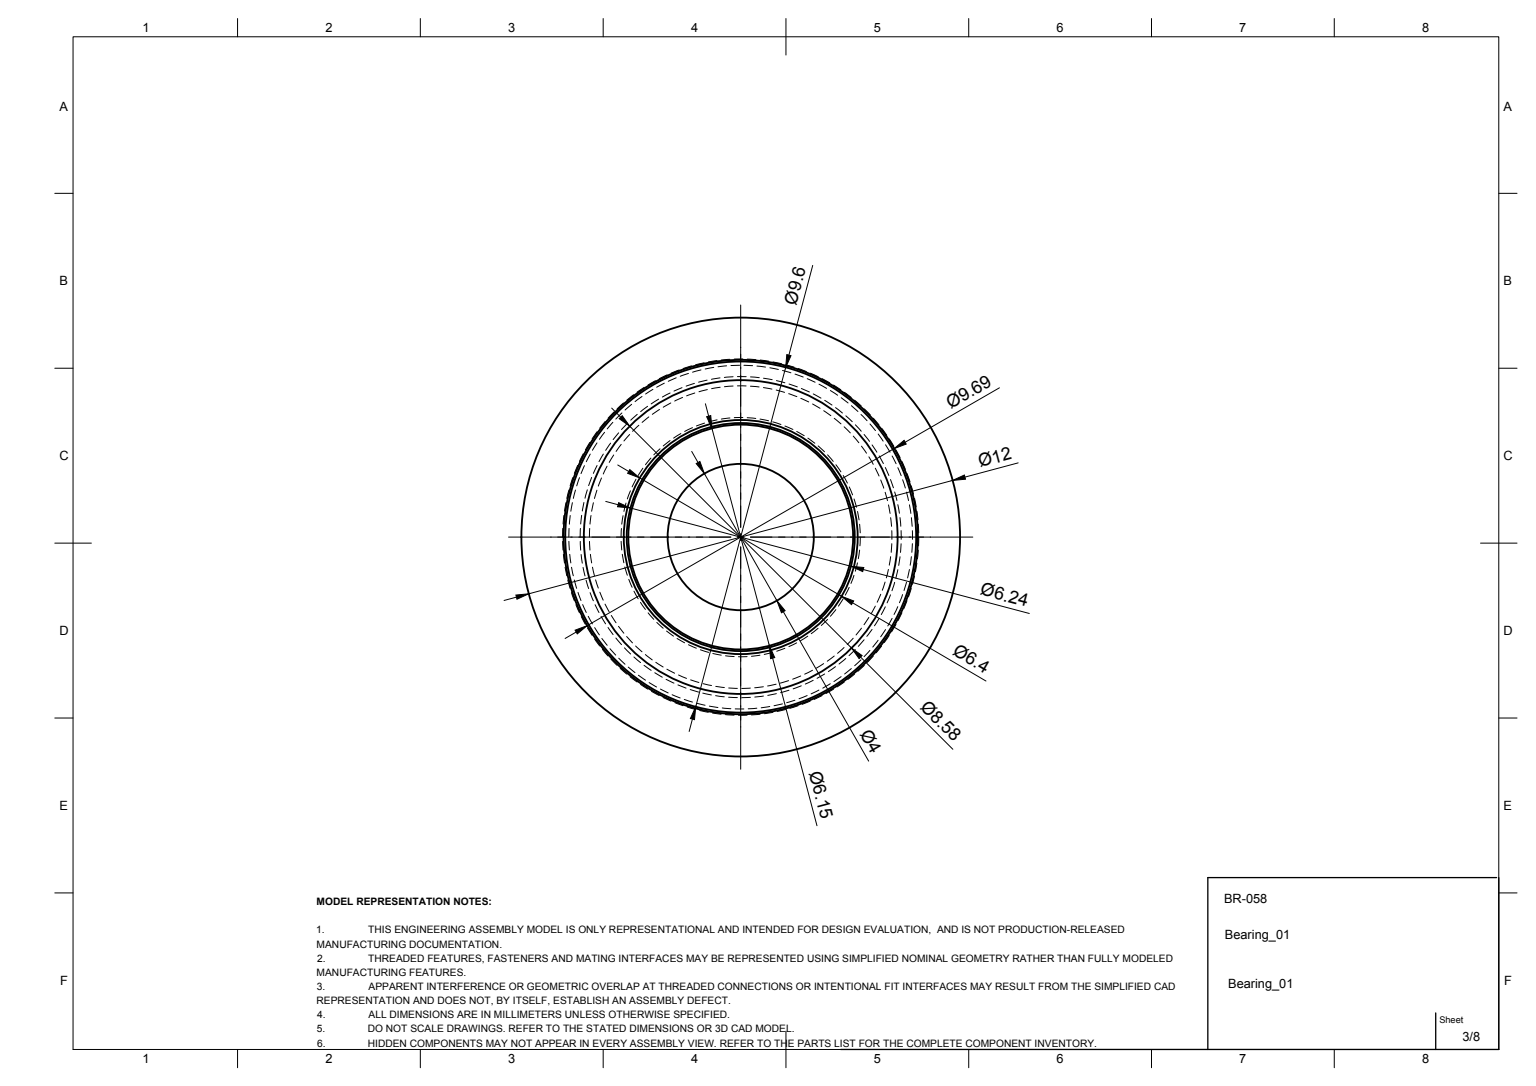
ISO-10303-21;
HEADER;
/* Generated by software containing ST-Developer
 * from STEP Tools, Inc. (www.steptools.com) 
 */

FILE_DESCRIPTION(
/* description */ (''),
/* implementation_level */ '2;1');

FILE_NAME(
/* name */ 'Bearing_01.step',
/* time_stamp */ '2026-10-12T16:07:47-07:00',
/* author */ (''),
/* organization */ (''),
/* preprocessor_version */ 'ST-DEVELOPER v20.2',
/* originating_system */ 'Autodesk Translation Framework v15.15.0.0',
/* authorisation */ '');

FILE_SCHEMA (('AUTOMOTIVE_DESIGN { 1 0 10303 214 3 1 1 }'));
ENDSEC;

DATA;
#10=MECHANICAL_DESIGN_GEOMETRIC_PRESENTATION_REPRESENTATION('',(#100,#101,#102,#103),#8779);
#43=CONICAL_SURFACE('',#5582,4.8,0.785398163397444);
#44=CONICAL_SURFACE('',#5593,4.845,0.785398163397444);
#45=CONICAL_SURFACE('',#5599,3.1184375,0.785398163397448);
#46=CONICAL_SURFACE('',#5617,3.0734375,0.785398163397448);
#47=CONICAL_SURFACE('',#5639,4.36638040039984,0.52359877559829);
#48=CONICAL_SURFACE('',#5648,4.57071796769724,1.04719755119659);
#49=CONICAL_SURFACE('',#5657,4.62071796769724,1.04719755119659);
#50=CONICAL_SURFACE('',#5666,4.27977786002139,0.52359877559829);
#51=CONICAL_SURFACE('',#5680,4.36638040039984,0.52359877559829);
#52=CONICAL_SURFACE('',#5689,4.57071796769724,1.04719755119659);
#53=CONICAL_SURFACE('',#5698,4.62071796769724,1.04719755119659);
#54=CONICAL_SURFACE('',#5707,4.27977786002139,0.52359877559829);
#56=TOROIDAL_SURFACE('',#5584,5.8,0.2);
#57=TOROIDAL_SURFACE('',#5590,5.8,0.2);
#58=TOROIDAL_SURFACE('',#5605,3.25741379310345,0.138976293103448);
#59=TOROIDAL_SURFACE('',#5611,3.25741379310345,0.138976293103448);
#60=TOROIDAL_SURFACE('',#5619,2.2,0.2);
#61=TOROIDAL_SURFACE('',#5625,2.2,0.2);
#62=TOROIDAL_SURFACE('',#5635,4.14313829631318,0.0900000000000005);
#63=TOROIDAL_SURFACE('',#5641,4.38370090847553,0.0200000000000002);
#64=TOROIDAL_SURFACE('',#5644,4.58,0.119999999999999);
#65=TOROIDAL_SURFACE('',#5650,4.51071796769724,0.12);
#66=TOROIDAL_SURFACE('',#5653,4.51071796769724,0.22);
#67=TOROIDAL_SURFACE('',#5659,4.58,0.219999999999999);
#68=TOROIDAL_SURFACE('',#5662,4.38370090847553,0.12);
#69=TOROIDAL_SURFACE('',#5676,4.14313829631318,0.0900000000000005);
#70=TOROIDAL_SURFACE('',#5682,4.38370090847553,0.0200000000000002);
#71=TOROIDAL_SURFACE('',#5685,4.58,0.119999999999999);
#72=TOROIDAL_SURFACE('',#5691,4.51071796769724,0.12);
#73=TOROIDAL_SURFACE('',#5694,4.51071796769724,0.22);
#74=TOROIDAL_SURFACE('',#5700,4.58,0.219999999999999);
#75=TOROIDAL_SURFACE('',#5703,4.38370090847553,0.12);
#86=SHAPE_REPRESENTATION_RELATIONSHIP('SRR','None',#8815,#93);
#93=ADVANCED_BREP_SHAPE_REPRESENTATION('',(#110,#111,#112,#113),#8778);
#100=STYLED_ITEM('',(#8856),#110);
#101=STYLED_ITEM('',(#8856),#111);
#102=STYLED_ITEM('',(#8856),#112);
#103=STYLED_ITEM('',(#8856),#113);
#110=MANIFOLD_SOLID_BREP('Body1',#5120);
#111=MANIFOLD_SOLID_BREP('Body2',#5121);
#112=MANIFOLD_SOLID_BREP('Body3',#5122);
#113=MANIFOLD_SOLID_BREP('Body4',#5123);
#151=FACE_BOUND('',#1015,.T.);
#152=FACE_BOUND('',#1017,.T.);
#153=FACE_BOUND('',#1019,.T.);
#154=FACE_BOUND('',#1021,.T.);
#155=FACE_BOUND('',#1033,.T.);
#156=FACE_BOUND('',#1035,.T.);
#157=FACE_BOUND('',#1037,.T.);
#158=FACE_BOUND('',#1039,.T.);
#159=FACE_BOUND('',#1053,.T.);
#160=FACE_BOUND('',#1055,.T.);
#161=FACE_BOUND('',#1057,.T.);
#162=FACE_BOUND('',#1059,.T.);
#163=FACE_BOUND('',#1061,.T.);
#164=FACE_BOUND('',#1075,.T.);
#165=FACE_BOUND('',#1077,.T.);
#166=FACE_BOUND('',#1079,.T.);
#167=FACE_BOUND('',#1081,.T.);
#168=FACE_BOUND('',#1083,.T.);
#314=CIRCLE('',#5573,4.8);
#315=CIRCLE('',#5574,4.8);
#316=CIRCLE('',#5576,4.872);
#317=CIRCLE('',#5577,4.872);
#318=CIRCLE('',#5579,4.8);
#319=CIRCLE('',#5580,4.8);
#320=CIRCLE('',#5581,4.8);
#321=CIRCLE('',#5583,4.845);
#322=CIRCLE('',#5585,6.);
#323=CIRCLE('',#5586,0.2);
#324=CIRCLE('',#5587,5.8);
#325=CIRCLE('',#5589,6.);
#326=CIRCLE('',#5591,5.8);
#327=CIRCLE('',#5592,0.2);
#328=CIRCLE('',#5594,4.845);
#329=CIRCLE('',#5600,3.1184375);
#330=CIRCLE('',#5601,3.0734375);
#331=CIRCLE('',#5602,3.1184375);
#332=CIRCLE('',#5604,3.1184375);
#333=CIRCLE('',#5606,0.138976293103448);
#334=CIRCLE('',#5607,3.2);
#335=CIRCLE('',#5609,3.272);
#336=CIRCLE('',#5610,3.272);
#337=CIRCLE('',#5612,3.2);
#338=CIRCLE('',#5613,0.138976293103448);
#339=CIRCLE('',#5614,3.1184375);
#340=CIRCLE('',#5616,3.1184375);
#341=CIRCLE('',#5618,3.0734375);
#342=CIRCLE('',#5620,2.2);
#343=CIRCLE('',#5621,0.2);
#344=CIRCLE('',#5622,2.);
#345=CIRCLE('',#5624,2.);
#346=CIRCLE('',#5626,0.2);
#347=CIRCLE('',#5627,2.2);
#348=CIRCLE('',#5633,3.2);
#349=CIRCLE('',#5634,3.2);
#350=CIRCLE('',#5636,4.22108058265378);
#351=CIRCLE('',#5637,0.0900000000000005);
#352=CIRCLE('',#5638,4.14313829631318);
#353=CIRCLE('',#5640,4.36638040039984);
#354=CIRCLE('',#5642,4.38370090847553);
#355=CIRCLE('',#5643,0.0200000000000002);
#356=CIRCLE('',#5645,4.64);
#357=CIRCLE('',#5646,0.119999999999999);
#358=CIRCLE('',#5647,4.58);
#359=CIRCLE('',#5649,4.57071796769724);
#360=CIRCLE('',#5651,4.39071796769724);
#361=CIRCLE('',#5652,0.12);
#362=CIRCLE('',#5654,4.62071796769724);
#363=CIRCLE('',#5655,0.22);
#364=CIRCLE('',#5656,4.29071796769724);
#365=CIRCLE('',#5658,4.69);
#366=CIRCLE('',#5660,4.58);
#367=CIRCLE('',#5661,0.219999999999999);
#368=CIRCLE('',#5663,4.27977786002139);
#369=CIRCLE('',#5664,0.12);
#370=CIRCLE('',#5665,4.38370090847553);
#371=CIRCLE('',#5667,4.13736479362129);
#372=CIRCLE('',#5674,3.2);
#373=CIRCLE('',#5675,3.2);
#374=CIRCLE('',#5677,4.22108058265378);
#375=CIRCLE('',#5678,0.0900000000000005);
#376=CIRCLE('',#5679,4.14313829631318);
#377=CIRCLE('',#5681,4.36638040039984);
#378=CIRCLE('',#5683,4.38370090847553);
#379=CIRCLE('',#5684,0.0200000000000002);
#380=CIRCLE('',#5686,4.64);
#381=CIRCLE('',#5687,0.119999999999999);
#382=CIRCLE('',#5688,4.58);
#383=CIRCLE('',#5690,4.57071796769724);
#384=CIRCLE('',#5692,4.39071796769724);
#385=CIRCLE('',#5693,0.12);
#386=CIRCLE('',#5695,4.62071796769724);
#387=CIRCLE('',#5696,0.22);
#388=CIRCLE('',#5697,4.29071796769724);
#389=CIRCLE('',#5699,4.69);
#390=CIRCLE('',#5701,4.58);
#391=CIRCLE('',#5702,0.219999999999999);
#392=CIRCLE('',#5704,4.27977786002139);
#393=CIRCLE('',#5705,0.12);
#394=CIRCLE('',#5706,4.38370090847553);
#395=CIRCLE('',#5708,4.13736479362129);
#465=CYLINDRICAL_SURFACE('',#5572,4.8);
#466=CYLINDRICAL_SURFACE('',#5575,4.872);
#467=CYLINDRICAL_SURFACE('',#5578,4.8);
#468=CYLINDRICAL_SURFACE('',#5588,6.);
#469=CYLINDRICAL_SURFACE('',#5603,3.1184375);
#470=CYLINDRICAL_SURFACE('',#5608,3.272);
#471=CYLINDRICAL_SURFACE('',#5615,3.1184375);
#472=CYLINDRICAL_SURFACE('',#5623,2.);
#473=CYLINDRICAL_SURFACE('',#5632,3.2);
#474=CYLINDRICAL_SURFACE('',#5673,3.2);
#692=FACE_OUTER_BOUND('',#1006,.T.);
#693=FACE_OUTER_BOUND('',#1007,.T.);
#694=FACE_OUTER_BOUND('',#1008,.T.);
#695=FACE_OUTER_BOUND('',#1009,.T.);
#696=FACE_OUTER_BOUND('',#1010,.T.);
#697=FACE_OUTER_BOUND('',#1011,.T.);
#698=FACE_OUTER_BOUND('',#1012,.T.);
#699=FACE_OUTER_BOUND('',#1013,.T.);
#700=FACE_OUTER_BOUND('',#1014,.T.);
#701=FACE_OUTER_BOUND('',#1016,.T.);
#702=FACE_OUTER_BOUND('',#1018,.T.);
#703=FACE_OUTER_BOUND('',#1020,.T.);
#704=FACE_OUTER_BOUND('',#1022,.T.);
#705=FACE_OUTER_BOUND('',#1023,.T.);
#706=FACE_OUTER_BOUND('',#1024,.T.);
#707=FACE_OUTER_BOUND('',#1025,.T.);
#708=FACE_OUTER_BOUND('',#1026,.T.);
#709=FACE_OUTER_BOUND('',#1027,.T.);
#710=FACE_OUTER_BOUND('',#1028,.T.);
#711=FACE_OUTER_BOUND('',#1029,.T.);
#712=FACE_OUTER_BOUND('',#1030,.T.);
#713=FACE_OUTER_BOUND('',#1031,.T.);
#714=FACE_OUTER_BOUND('',#1032,.T.);
#715=FACE_OUTER_BOUND('',#1034,.T.);
#716=FACE_OUTER_BOUND('',#1036,.T.);
#717=FACE_OUTER_BOUND('',#1038,.T.);
#718=FACE_OUTER_BOUND('',#1040,.T.);
#719=FACE_OUTER_BOUND('',#1041,.T.);
#720=FACE_OUTER_BOUND('',#1042,.T.);
#721=FACE_OUTER_BOUND('',#1043,.T.);
#722=FACE_OUTER_BOUND('',#1044,.T.);
#723=FACE_OUTER_BOUND('',#1045,.T.);
#724=FACE_OUTER_BOUND('',#1046,.T.);
#725=FACE_OUTER_BOUND('',#1047,.T.);
#726=FACE_OUTER_BOUND('',#1048,.T.);
#727=FACE_OUTER_BOUND('',#1049,.T.);
#728=FACE_OUTER_BOUND('',#1050,.T.);
#729=FACE_OUTER_BOUND('',#1051,.T.);
#730=FACE_OUTER_BOUND('',#1052,.T.);
#731=FACE_OUTER_BOUND('',#1054,.T.);
#732=FACE_OUTER_BOUND('',#1056,.T.);
#733=FACE_OUTER_BOUND('',#1058,.T.);
#734=FACE_OUTER_BOUND('',#1060,.T.);
#735=FACE_OUTER_BOUND('',#1062,.T.);
#736=FACE_OUTER_BOUND('',#1063,.T.);
#737=FACE_OUTER_BOUND('',#1064,.T.);
#738=FACE_OUTER_BOUND('',#1065,.T.);
#739=FACE_OUTER_BOUND('',#1066,.T.);
#740=FACE_OUTER_BOUND('',#1067,.T.);
#741=FACE_OUTER_BOUND('',#1068,.T.);
#742=FACE_OUTER_BOUND('',#1069,.T.);
#743=FACE_OUTER_BOUND('',#1070,.T.);
#744=FACE_OUTER_BOUND('',#1071,.T.);
#745=FACE_OUTER_BOUND('',#1072,.T.);
#746=FACE_OUTER_BOUND('',#1073,.T.);
#747=FACE_OUTER_BOUND('',#1074,.T.);
#748=FACE_OUTER_BOUND('',#1076,.T.);
#749=FACE_OUTER_BOUND('',#1078,.T.);
#750=FACE_OUTER_BOUND('',#1080,.T.);
#751=FACE_OUTER_BOUND('',#1082,.T.);
#1006=EDGE_LOOP('',(#4464,#4465,#4466,#4467));
#1007=EDGE_LOOP('',(#4468,#4469,#4470,#4471));
#1008=EDGE_LOOP('',(#4472,#4473,#4474,#4475,#4476));
#1009=EDGE_LOOP('',(#4477,#4478,#4479,#4480,#4481));
#1010=EDGE_LOOP('',(#4482,#4483,#4484,#4485));
#1011=EDGE_LOOP('',(#4486,#4487,#4488,#4489));
#1012=EDGE_LOOP('',(#4490,#4491,#4492,#4493));
#1013=EDGE_LOOP('',(#4494,#4495,#4496,#4497));
#1014=EDGE_LOOP('',(#4498));
#1015=EDGE_LOOP('',(#4499));
#1016=EDGE_LOOP('',(#4500));
#1017=EDGE_LOOP('',(#4501));
#1018=EDGE_LOOP('',(#4502));
#1019=EDGE_LOOP('',(#4503));
#1020=EDGE_LOOP('',(#4504));
#1021=EDGE_LOOP('',(#4505));
#1022=EDGE_LOOP('',(#4506,#4507,#4508,#4509,#4510));
#1023=EDGE_LOOP('',(#4511,#4512,#4513,#4514,#4515));
#1024=EDGE_LOOP('',(#4516,#4517,#4518,#4519));
#1025=EDGE_LOOP('',(#4520,#4521,#4522,#4523));
#1026=EDGE_LOOP('',(#4524,#4525,#4526,#4527));
#1027=EDGE_LOOP('',(#4528,#4529,#4530,#4531));
#1028=EDGE_LOOP('',(#4532,#4533,#4534,#4535));
#1029=EDGE_LOOP('',(#4536,#4537,#4538,#4539));
#1030=EDGE_LOOP('',(#4540,#4541,#4542,#4543));
#1031=EDGE_LOOP('',(#4544,#4545,#4546,#4547));
#1032=EDGE_LOOP('',(#4548));
#1033=EDGE_LOOP('',(#4549));
#1034=EDGE_LOOP('',(#4550));
#1035=EDGE_LOOP('',(#4551));
#1036=EDGE_LOOP('',(#4552));
#1037=EDGE_LOOP('',(#4553));
#1038=EDGE_LOOP('',(#4554));
#1039=EDGE_LOOP('',(#4555));
#1040=EDGE_LOOP('',(#4556,#4557,#4558,#4559));
#1041=EDGE_LOOP('',(#4560,#4561,#4562,#4563));
#1042=EDGE_LOOP('',(#4564,#4565,#4566,#4567));
#1043=EDGE_LOOP('',(#4568,#4569,#4570,#4571));
#1044=EDGE_LOOP('',(#4572,#4573,#4574,#4575));
#1045=EDGE_LOOP('',(#4576,#4577,#4578,#4579));
#1046=EDGE_LOOP('',(#4580,#4581,#4582,#4583));
#1047=EDGE_LOOP('',(#4584,#4585,#4586,#4587));
#1048=EDGE_LOOP('',(#4588,#4589,#4590,#4591));
#1049=EDGE_LOOP('',(#4592,#4593,#4594,#4595));
#1050=EDGE_LOOP('',(#4596,#4597,#4598,#4599));
#1051=EDGE_LOOP('',(#4600,#4601,#4602,#4603));
#1052=EDGE_LOOP('',(#4604));
#1053=EDGE_LOOP('',(#4605));
#1054=EDGE_LOOP('',(#4606));
#1055=EDGE_LOOP('',(#4607));
#1056=EDGE_LOOP('',(#4608));
#1057=EDGE_LOOP('',(#4609));
#1058=EDGE_LOOP('',(#4610));
#1059=EDGE_LOOP('',(#4611));
#1060=EDGE_LOOP('',(#4612));
#1061=EDGE_LOOP('',(#4613));
#1062=EDGE_LOOP('',(#4614,#4615,#4616,#4617));
#1063=EDGE_LOOP('',(#4618,#4619,#4620,#4621));
#1064=EDGE_LOOP('',(#4622,#4623,#4624,#4625));
#1065=EDGE_LOOP('',(#4626,#4627,#4628,#4629));
#1066=EDGE_LOOP('',(#4630,#4631,#4632,#4633));
#1067=EDGE_LOOP('',(#4634,#4635,#4636,#4637));
#1068=EDGE_LOOP('',(#4638,#4639,#4640,#4641));
#1069=EDGE_LOOP('',(#4642,#4643,#4644,#4645));
#1070=EDGE_LOOP('',(#4646,#4647,#4648,#4649));
#1071=EDGE_LOOP('',(#4650,#4651,#4652,#4653));
#1072=EDGE_LOOP('',(#4654,#4655,#4656,#4657));
#1073=EDGE_LOOP('',(#4658,#4659,#4660,#4661));
#1074=EDGE_LOOP('',(#4662));
#1075=EDGE_LOOP('',(#4663));
#1076=EDGE_LOOP('',(#4664));
#1077=EDGE_LOOP('',(#4665));
#1078=EDGE_LOOP('',(#4666));
#1079=EDGE_LOOP('',(#4667));
#1080=EDGE_LOOP('',(#4668));
#1081=EDGE_LOOP('',(#4669));
#1082=EDGE_LOOP('',(#4670));
#1083=EDGE_LOOP('',(#4671));
#1547=LINE('',#8532,#2032);
#1548=LINE('',#8538,#2033);
#1549=LINE('',#8546,#2034);
#1550=LINE('',#8550,#2035);
#1551=LINE('',#8561,#2036);
#1552=LINE('',#8568,#2037);
#1553=LINE('',#8579,#2038);
#1554=LINE('',#8584,#2039);
#1555=LINE('',#8594,#2040);
#1556=LINE('',#8604,#2041);
#1557=LINE('',#8608,#2042);
#1558=LINE('',#8618,#2043);
#1559=LINE('',#8632,#2044);
#1560=LINE('',#8643,#2045);
#1561=LINE('',#8657,#2046);
#1562=LINE('',#8671,#2047);
#1563=LINE('',#8685,#2048);
#1564=LINE('',#8695,#2049);
#1565=LINE('',#8706,#2050);
#1566=LINE('',#8720,#2051);
#1567=LINE('',#8734,#2052);
#1568=LINE('',#8748,#2053);
#2032=VECTOR('',#6929,4.8);
#2033=VECTOR('',#6936,4.872);
#2034=VECTOR('',#6945,4.8);
#2035=VECTOR('',#6950,4.8);
#2036=VECTOR('',#6965,6.);
#2037=VECTOR('',#6974,4.845);
#2038=VECTOR('',#6989,3.1184375);
#2039=VECTOR('',#6996,3.1184375);
#2040=VECTOR('',#7009,3.272);
#2041=VECTOR('',#7022,3.1184375);
#2042=VECTOR('',#7027,3.0734375);
#2043=VECTOR('',#7040,2.);
#2044=VECTOR('',#7061,3.2);
#2045=VECTOR('',#7076,4.36638040039984);
#2046=VECTOR('',#7095,4.57071796769724);
#2047=VECTOR('',#7114,4.62071796769724);
#2048=VECTOR('',#7133,4.27977786002139);
#2049=VECTOR('',#7148,3.2);
#2050=VECTOR('',#7163,4.36638040039984);
#2051=VECTOR('',#7182,4.57071796769724);
#2052=VECTOR('',#7201,4.62071796769724);
#2053=VECTOR('',#7220,4.27977786002139);
#2462=VERTEX_POINT('',#8529);
#2463=VERTEX_POINT('',#8531);
#2464=VERTEX_POINT('',#8535);
#2465=VERTEX_POINT('',#8537);
#2466=VERTEX_POINT('',#8541);
#2467=VERTEX_POINT('',#8542);
#2468=VERTEX_POINT('',#8545);
#2469=VERTEX_POINT('',#8549);
#2470=VERTEX_POINT('',#8553);
#2471=VERTEX_POINT('',#8555);
#2472=VERTEX_POINT('',#8559);
#2473=VERTEX_POINT('',#8563);
#2474=VERTEX_POINT('',#8567);
#2475=VERTEX_POINT('',#8575);
#2476=VERTEX_POINT('',#8576);
#2477=VERTEX_POINT('',#8578);
#2478=VERTEX_POINT('',#8583);
#2479=VERTEX_POINT('',#8587);
#2480=VERTEX_POINT('',#8591);
#2481=VERTEX_POINT('',#8593);
#2482=VERTEX_POINT('',#8597);
#2483=VERTEX_POINT('',#8599);
#2484=VERTEX_POINT('',#8603);
#2485=VERTEX_POINT('',#8607);
#2486=VERTEX_POINT('',#8611);
#2487=VERTEX_POINT('',#8613);
#2488=VERTEX_POINT('',#8617);
#2489=VERTEX_POINT('',#8621);
#2490=VERTEX_POINT('',#8629);
#2491=VERTEX_POINT('',#8631);
#2492=VERTEX_POINT('',#8635);
#2493=VERTEX_POINT('',#8637);
#2494=VERTEX_POINT('',#8641);
#2495=VERTEX_POINT('',#8645);
#2496=VERTEX_POINT('',#8649);
#2497=VERTEX_POINT('',#8651);
#2498=VERTEX_POINT('',#8655);
#2499=VERTEX_POINT('',#8659);
#2500=VERTEX_POINT('',#8663);
#2501=VERTEX_POINT('',#8665);
#2502=VERTEX_POINT('',#8669);
#2503=VERTEX_POINT('',#8673);
#2504=VERTEX_POINT('',#8677);
#2505=VERTEX_POINT('',#8679);
#2506=VERTEX_POINT('',#8683);
#2507=VERTEX_POINT('',#8692);
#2508=VERTEX_POINT('',#8694);
#2509=VERTEX_POINT('',#8698);
#2510=VERTEX_POINT('',#8700);
#2511=VERTEX_POINT('',#8704);
#2512=VERTEX_POINT('',#8708);
#2513=VERTEX_POINT('',#8712);
#2514=VERTEX_POINT('',#8714);
#2515=VERTEX_POINT('',#8718);
#2516=VERTEX_POINT('',#8722);
#2517=VERTEX_POINT('',#8726);
#2518=VERTEX_POINT('',#8728);
#2519=VERTEX_POINT('',#8732);
#2520=VERTEX_POINT('',#8736);
#2521=VERTEX_POINT('',#8740);
#2522=VERTEX_POINT('',#8742);
#2523=VERTEX_POINT('',#8746);
#3136=EDGE_CURVE('',#2462,#2462,#314,.T.);
#3137=EDGE_CURVE('',#2462,#2463,#1547,.T.);
#3138=EDGE_CURVE('',#2463,#2463,#315,.T.);
#3139=EDGE_CURVE('',#2464,#2464,#316,.T.);
#3140=EDGE_CURVE('',#2464,#2465,#1548,.T.);
#3141=EDGE_CURVE('',#2465,#2465,#317,.T.);
#3142=EDGE_CURVE('',#2466,#2467,#318,.T.);
#3143=EDGE_CURVE('',#2467,#2466,#319,.T.);
#3144=EDGE_CURVE('',#2467,#2468,#1549,.T.);
#3145=EDGE_CURVE('',#2468,#2468,#320,.T.);
#3146=EDGE_CURVE('',#2466,#2469,#1550,.T.);
#3147=EDGE_CURVE('',#2469,#2469,#321,.T.);
#3148=EDGE_CURVE('',#2470,#2470,#322,.T.);
#3149=EDGE_CURVE('',#2470,#2471,#323,.T.);
#3150=EDGE_CURVE('',#2471,#2471,#324,.T.);
#3151=EDGE_CURVE('',#2472,#2472,#325,.T.);
#3152=EDGE_CURVE('',#2472,#2470,#1551,.T.);
#3153=EDGE_CURVE('',#2473,#2473,#326,.T.);
#3154=EDGE_CURVE('',#2473,#2472,#327,.T.);
#3155=EDGE_CURVE('',#2463,#2474,#1552,.T.);
#3156=EDGE_CURVE('',#2474,#2474,#328,.T.);
#3157=EDGE_CURVE('',#2475,#2476,#329,.T.);
#3158=EDGE_CURVE('',#2476,#2477,#1553,.T.);
#3159=EDGE_CURVE('',#2477,#2477,#330,.T.);
#3160=EDGE_CURVE('',#2476,#2475,#331,.T.);
#3161=EDGE_CURVE('',#2475,#2478,#1554,.T.);
#3162=EDGE_CURVE('',#2478,#2478,#332,.T.);
#3163=EDGE_CURVE('',#2478,#2479,#333,.T.);
#3164=EDGE_CURVE('',#2479,#2479,#334,.T.);
#3165=EDGE_CURVE('',#2480,#2480,#335,.T.);
#3166=EDGE_CURVE('',#2480,#2481,#1555,.T.);
#3167=EDGE_CURVE('',#2481,#2481,#336,.T.);
#3168=EDGE_CURVE('',#2482,#2482,#337,.T.);
#3169=EDGE_CURVE('',#2482,#2483,#338,.T.);
#3170=EDGE_CURVE('',#2483,#2483,#339,.T.);
#3171=EDGE_CURVE('',#2483,#2484,#1556,.T.);
#3172=EDGE_CURVE('',#2484,#2484,#340,.T.);
#3173=EDGE_CURVE('',#2484,#2485,#1557,.T.);
#3174=EDGE_CURVE('',#2485,#2485,#341,.T.);
#3175=EDGE_CURVE('',#2486,#2486,#342,.T.);
#3176=EDGE_CURVE('',#2486,#2487,#343,.T.);
#3177=EDGE_CURVE('',#2487,#2487,#344,.T.);
#3178=EDGE_CURVE('',#2487,#2488,#1558,.T.);
#3179=EDGE_CURVE('',#2488,#2488,#345,.T.);
#3180=EDGE_CURVE('',#2488,#2489,#346,.T.);
#3181=EDGE_CURVE('',#2489,#2489,#347,.T.);
#3182=EDGE_CURVE('',#2490,#2490,#348,.T.);
#3183=EDGE_CURVE('',#2490,#2491,#1559,.T.);
#3184=EDGE_CURVE('',#2491,#2491,#349,.T.);
#3185=EDGE_CURVE('',#2492,#2492,#350,.T.);
#3186=EDGE_CURVE('',#2492,#2493,#351,.T.);
#3187=EDGE_CURVE('',#2493,#2493,#352,.T.);
#3188=EDGE_CURVE('',#2494,#2494,#353,.T.);
#3189=EDGE_CURVE('',#2494,#2492,#1560,.T.);
#3190=EDGE_CURVE('',#2495,#2495,#354,.T.);
#3191=EDGE_CURVE('',#2495,#2494,#355,.T.);
#3192=EDGE_CURVE('',#2496,#2496,#356,.T.);
#3193=EDGE_CURVE('',#2496,#2497,#357,.T.);
#3194=EDGE_CURVE('',#2497,#2497,#358,.T.);
#3195=EDGE_CURVE('',#2498,#2498,#359,.T.);
#3196=EDGE_CURVE('',#2498,#2496,#1561,.T.);
#3197=EDGE_CURVE('',#2499,#2499,#360,.T.);
#3198=EDGE_CURVE('',#2499,#2498,#361,.T.);
#3199=EDGE_CURVE('',#2500,#2500,#362,.T.);
#3200=EDGE_CURVE('',#2500,#2501,#363,.T.);
#3201=EDGE_CURVE('',#2501,#2501,#364,.T.);
#3202=EDGE_CURVE('',#2502,#2502,#365,.T.);
#3203=EDGE_CURVE('',#2502,#2500,#1562,.T.);
#3204=EDGE_CURVE('',#2503,#2503,#366,.T.);
#3205=EDGE_CURVE('',#2503,#2502,#367,.T.);
#3206=EDGE_CURVE('',#2504,#2504,#368,.T.);
#3207=EDGE_CURVE('',#2504,#2505,#369,.T.);
#3208=EDGE_CURVE('',#2505,#2505,#370,.T.);
#3209=EDGE_CURVE('',#2506,#2506,#371,.T.);
#3210=EDGE_CURVE('',#2506,#2504,#1563,.T.);
#3211=EDGE_CURVE('',#2507,#2507,#372,.T.);
#3212=EDGE_CURVE('',#2507,#2508,#1564,.T.);
#3213=EDGE_CURVE('',#2508,#2508,#373,.T.);
#3214=EDGE_CURVE('',#2509,#2509,#374,.T.);
#3215=EDGE_CURVE('',#2509,#2510,#375,.T.);
#3216=EDGE_CURVE('',#2510,#2510,#376,.T.);
#3217=EDGE_CURVE('',#2511,#2511,#377,.T.);
#3218=EDGE_CURVE('',#2511,#2509,#1565,.T.);
#3219=EDGE_CURVE('',#2512,#2512,#378,.T.);
#3220=EDGE_CURVE('',#2512,#2511,#379,.T.);
#3221=EDGE_CURVE('',#2513,#2513,#380,.T.);
#3222=EDGE_CURVE('',#2513,#2514,#381,.T.);
#3223=EDGE_CURVE('',#2514,#2514,#382,.T.);
#3224=EDGE_CURVE('',#2515,#2515,#383,.T.);
#3225=EDGE_CURVE('',#2515,#2513,#1566,.T.);
#3226=EDGE_CURVE('',#2516,#2516,#384,.T.);
#3227=EDGE_CURVE('',#2516,#2515,#385,.T.);
#3228=EDGE_CURVE('',#2517,#2517,#386,.T.);
#3229=EDGE_CURVE('',#2517,#2518,#387,.T.);
#3230=EDGE_CURVE('',#2518,#2518,#388,.T.);
#3231=EDGE_CURVE('',#2519,#2519,#389,.T.);
#3232=EDGE_CURVE('',#2519,#2517,#1567,.T.);
#3233=EDGE_CURVE('',#2520,#2520,#390,.T.);
#3234=EDGE_CURVE('',#2520,#2519,#391,.T.);
#3235=EDGE_CURVE('',#2521,#2521,#392,.T.);
#3236=EDGE_CURVE('',#2521,#2522,#393,.T.);
#3237=EDGE_CURVE('',#2522,#2522,#394,.T.);
#3238=EDGE_CURVE('',#2523,#2523,#395,.T.);
#3239=EDGE_CURVE('',#2523,#2521,#1568,.T.);
#4464=ORIENTED_EDGE('',*,*,#3136,.F.);
#4465=ORIENTED_EDGE('',*,*,#3137,.T.);
#4466=ORIENTED_EDGE('',*,*,#3138,.T.);
#4467=ORIENTED_EDGE('',*,*,#3137,.F.);
#4468=ORIENTED_EDGE('',*,*,#3139,.F.);
#4469=ORIENTED_EDGE('',*,*,#3140,.T.);
#4470=ORIENTED_EDGE('',*,*,#3141,.T.);
#4471=ORIENTED_EDGE('',*,*,#3140,.F.);
#4472=ORIENTED_EDGE('',*,*,#3142,.F.);
#4473=ORIENTED_EDGE('',*,*,#3143,.F.);
#4474=ORIENTED_EDGE('',*,*,#3144,.T.);
#4475=ORIENTED_EDGE('',*,*,#3145,.T.);
#4476=ORIENTED_EDGE('',*,*,#3144,.F.);
#4477=ORIENTED_EDGE('',*,*,#3142,.T.);
#4478=ORIENTED_EDGE('',*,*,#3143,.T.);
#4479=ORIENTED_EDGE('',*,*,#3146,.T.);
#4480=ORIENTED_EDGE('',*,*,#3147,.F.);
#4481=ORIENTED_EDGE('',*,*,#3146,.F.);
#4482=ORIENTED_EDGE('',*,*,#3148,.F.);
#4483=ORIENTED_EDGE('',*,*,#3149,.T.);
#4484=ORIENTED_EDGE('',*,*,#3150,.T.);
#4485=ORIENTED_EDGE('',*,*,#3149,.F.);
#4486=ORIENTED_EDGE('',*,*,#3151,.F.);
#4487=ORIENTED_EDGE('',*,*,#3152,.T.);
#4488=ORIENTED_EDGE('',*,*,#3148,.T.);
#4489=ORIENTED_EDGE('',*,*,#3152,.F.);
#4490=ORIENTED_EDGE('',*,*,#3153,.F.);
#4491=ORIENTED_EDGE('',*,*,#3154,.T.);
#4492=ORIENTED_EDGE('',*,*,#3151,.T.);
#4493=ORIENTED_EDGE('',*,*,#3154,.F.);
#4494=ORIENTED_EDGE('',*,*,#3138,.F.);
#4495=ORIENTED_EDGE('',*,*,#3155,.T.);
#4496=ORIENTED_EDGE('',*,*,#3156,.T.);
#4497=ORIENTED_EDGE('',*,*,#3155,.F.);
#4498=ORIENTED_EDGE('',*,*,#3153,.T.);
#4499=ORIENTED_EDGE('',*,*,#3156,.F.);
#4500=ORIENTED_EDGE('',*,*,#3150,.F.);
#4501=ORIENTED_EDGE('',*,*,#3147,.T.);
#4502=ORIENTED_EDGE('',*,*,#3139,.T.);
#4503=ORIENTED_EDGE('',*,*,#3145,.F.);
#4504=ORIENTED_EDGE('',*,*,#3141,.F.);
#4505=ORIENTED_EDGE('',*,*,#3136,.T.);
#4506=ORIENTED_EDGE('',*,*,#3157,.T.);
#4507=ORIENTED_EDGE('',*,*,#3158,.T.);
#4508=ORIENTED_EDGE('',*,*,#3159,.F.);
#4509=ORIENTED_EDGE('',*,*,#3158,.F.);
#4510=ORIENTED_EDGE('',*,*,#3160,.T.);
#4511=ORIENTED_EDGE('',*,*,#3157,.F.);
#4512=ORIENTED_EDGE('',*,*,#3161,.T.);
#4513=ORIENTED_EDGE('',*,*,#3162,.T.);
#4514=ORIENTED_EDGE('',*,*,#3161,.F.);
#4515=ORIENTED_EDGE('',*,*,#3160,.F.);
#4516=ORIENTED_EDGE('',*,*,#3162,.F.);
#4517=ORIENTED_EDGE('',*,*,#3163,.T.);
#4518=ORIENTED_EDGE('',*,*,#3164,.T.);
#4519=ORIENTED_EDGE('',*,*,#3163,.F.);
#4520=ORIENTED_EDGE('',*,*,#3165,.F.);
#4521=ORIENTED_EDGE('',*,*,#3166,.T.);
#4522=ORIENTED_EDGE('',*,*,#3167,.T.);
#4523=ORIENTED_EDGE('',*,*,#3166,.F.);
#4524=ORIENTED_EDGE('',*,*,#3168,.F.);
#4525=ORIENTED_EDGE('',*,*,#3169,.T.);
#4526=ORIENTED_EDGE('',*,*,#3170,.T.);
#4527=ORIENTED_EDGE('',*,*,#3169,.F.);
#4528=ORIENTED_EDGE('',*,*,#3170,.F.);
#4529=ORIENTED_EDGE('',*,*,#3171,.T.);
#4530=ORIENTED_EDGE('',*,*,#3172,.T.);
#4531=ORIENTED_EDGE('',*,*,#3171,.F.);
#4532=ORIENTED_EDGE('',*,*,#3172,.F.);
#4533=ORIENTED_EDGE('',*,*,#3173,.T.);
#4534=ORIENTED_EDGE('',*,*,#3174,.T.);
#4535=ORIENTED_EDGE('',*,*,#3173,.F.);
#4536=ORIENTED_EDGE('',*,*,#3175,.F.);
#4537=ORIENTED_EDGE('',*,*,#3176,.T.);
#4538=ORIENTED_EDGE('',*,*,#3177,.T.);
#4539=ORIENTED_EDGE('',*,*,#3176,.F.);
#4540=ORIENTED_EDGE('',*,*,#3177,.F.);
#4541=ORIENTED_EDGE('',*,*,#3178,.T.);
#4542=ORIENTED_EDGE('',*,*,#3179,.T.);
#4543=ORIENTED_EDGE('',*,*,#3178,.F.);
#4544=ORIENTED_EDGE('',*,*,#3179,.F.);
#4545=ORIENTED_EDGE('',*,*,#3180,.T.);
#4546=ORIENTED_EDGE('',*,*,#3181,.T.);
#4547=ORIENTED_EDGE('',*,*,#3180,.F.);
#4548=ORIENTED_EDGE('',*,*,#3174,.F.);
#4549=ORIENTED_EDGE('',*,*,#3175,.T.);
#4550=ORIENTED_EDGE('',*,*,#3167,.F.);
#4551=ORIENTED_EDGE('',*,*,#3168,.T.);
#4552=ORIENTED_EDGE('',*,*,#3165,.T.);
#4553=ORIENTED_EDGE('',*,*,#3164,.F.);
#4554=ORIENTED_EDGE('',*,*,#3159,.T.);
#4555=ORIENTED_EDGE('',*,*,#3181,.F.);
#4556=ORIENTED_EDGE('',*,*,#3182,.F.);
#4557=ORIENTED_EDGE('',*,*,#3183,.T.);
#4558=ORIENTED_EDGE('',*,*,#3184,.T.);
#4559=ORIENTED_EDGE('',*,*,#3183,.F.);
#4560=ORIENTED_EDGE('',*,*,#3185,.F.);
#4561=ORIENTED_EDGE('',*,*,#3186,.T.);
#4562=ORIENTED_EDGE('',*,*,#3187,.T.);
#4563=ORIENTED_EDGE('',*,*,#3186,.F.);
#4564=ORIENTED_EDGE('',*,*,#3188,.F.);
#4565=ORIENTED_EDGE('',*,*,#3189,.T.);
#4566=ORIENTED_EDGE('',*,*,#3185,.T.);
#4567=ORIENTED_EDGE('',*,*,#3189,.F.);
#4568=ORIENTED_EDGE('',*,*,#3190,.F.);
#4569=ORIENTED_EDGE('',*,*,#3191,.T.);
#4570=ORIENTED_EDGE('',*,*,#3188,.T.);
#4571=ORIENTED_EDGE('',*,*,#3191,.F.);
#4572=ORIENTED_EDGE('',*,*,#3192,.F.);
#4573=ORIENTED_EDGE('',*,*,#3193,.T.);
#4574=ORIENTED_EDGE('',*,*,#3194,.T.);
#4575=ORIENTED_EDGE('',*,*,#3193,.F.);
#4576=ORIENTED_EDGE('',*,*,#3195,.F.);
#4577=ORIENTED_EDGE('',*,*,#3196,.T.);
#4578=ORIENTED_EDGE('',*,*,#3192,.T.);
#4579=ORIENTED_EDGE('',*,*,#3196,.F.);
#4580=ORIENTED_EDGE('',*,*,#3197,.F.);
#4581=ORIENTED_EDGE('',*,*,#3198,.T.);
#4582=ORIENTED_EDGE('',*,*,#3195,.T.);
#4583=ORIENTED_EDGE('',*,*,#3198,.F.);
#4584=ORIENTED_EDGE('',*,*,#3199,.F.);
#4585=ORIENTED_EDGE('',*,*,#3200,.T.);
#4586=ORIENTED_EDGE('',*,*,#3201,.T.);
#4587=ORIENTED_EDGE('',*,*,#3200,.F.);
#4588=ORIENTED_EDGE('',*,*,#3202,.F.);
#4589=ORIENTED_EDGE('',*,*,#3203,.T.);
#4590=ORIENTED_EDGE('',*,*,#3199,.T.);
#4591=ORIENTED_EDGE('',*,*,#3203,.F.);
#4592=ORIENTED_EDGE('',*,*,#3204,.F.);
#4593=ORIENTED_EDGE('',*,*,#3205,.T.);
#4594=ORIENTED_EDGE('',*,*,#3202,.T.);
#4595=ORIENTED_EDGE('',*,*,#3205,.F.);
#4596=ORIENTED_EDGE('',*,*,#3206,.F.);
#4597=ORIENTED_EDGE('',*,*,#3207,.T.);
#4598=ORIENTED_EDGE('',*,*,#3208,.T.);
#4599=ORIENTED_EDGE('',*,*,#3207,.F.);
#4600=ORIENTED_EDGE('',*,*,#3209,.F.);
#4601=ORIENTED_EDGE('',*,*,#3210,.T.);
#4602=ORIENTED_EDGE('',*,*,#3206,.T.);
#4603=ORIENTED_EDGE('',*,*,#3210,.F.);
#4604=ORIENTED_EDGE('',*,*,#3209,.T.);
#4605=ORIENTED_EDGE('',*,*,#3184,.F.);
#4606=ORIENTED_EDGE('',*,*,#3204,.T.);
#4607=ORIENTED_EDGE('',*,*,#3208,.F.);
#4608=ORIENTED_EDGE('',*,*,#3197,.T.);
#4609=ORIENTED_EDGE('',*,*,#3201,.F.);
#4610=ORIENTED_EDGE('',*,*,#3194,.F.);
#4611=ORIENTED_EDGE('',*,*,#3190,.T.);
#4612=ORIENTED_EDGE('',*,*,#3187,.F.);
#4613=ORIENTED_EDGE('',*,*,#3182,.T.);
#4614=ORIENTED_EDGE('',*,*,#3211,.T.);
#4615=ORIENTED_EDGE('',*,*,#3212,.T.);
#4616=ORIENTED_EDGE('',*,*,#3213,.F.);
#4617=ORIENTED_EDGE('',*,*,#3212,.F.);
#4618=ORIENTED_EDGE('',*,*,#3214,.T.);
#4619=ORIENTED_EDGE('',*,*,#3215,.T.);
#4620=ORIENTED_EDGE('',*,*,#3216,.F.);
#4621=ORIENTED_EDGE('',*,*,#3215,.F.);
#4622=ORIENTED_EDGE('',*,*,#3217,.T.);
#4623=ORIENTED_EDGE('',*,*,#3218,.T.);
#4624=ORIENTED_EDGE('',*,*,#3214,.F.);
#4625=ORIENTED_EDGE('',*,*,#3218,.F.);
#4626=ORIENTED_EDGE('',*,*,#3219,.T.);
#4627=ORIENTED_EDGE('',*,*,#3220,.T.);
#4628=ORIENTED_EDGE('',*,*,#3217,.F.);
#4629=ORIENTED_EDGE('',*,*,#3220,.F.);
#4630=ORIENTED_EDGE('',*,*,#3221,.T.);
#4631=ORIENTED_EDGE('',*,*,#3222,.T.);
#4632=ORIENTED_EDGE('',*,*,#3223,.F.);
#4633=ORIENTED_EDGE('',*,*,#3222,.F.);
#4634=ORIENTED_EDGE('',*,*,#3224,.T.);
#4635=ORIENTED_EDGE('',*,*,#3225,.T.);
#4636=ORIENTED_EDGE('',*,*,#3221,.F.);
#4637=ORIENTED_EDGE('',*,*,#3225,.F.);
#4638=ORIENTED_EDGE('',*,*,#3226,.T.);
#4639=ORIENTED_EDGE('',*,*,#3227,.T.);
#4640=ORIENTED_EDGE('',*,*,#3224,.F.);
#4641=ORIENTED_EDGE('',*,*,#3227,.F.);
#4642=ORIENTED_EDGE('',*,*,#3228,.T.);
#4643=ORIENTED_EDGE('',*,*,#3229,.T.);
#4644=ORIENTED_EDGE('',*,*,#3230,.F.);
#4645=ORIENTED_EDGE('',*,*,#3229,.F.);
#4646=ORIENTED_EDGE('',*,*,#3231,.T.);
#4647=ORIENTED_EDGE('',*,*,#3232,.T.);
#4648=ORIENTED_EDGE('',*,*,#3228,.F.);
#4649=ORIENTED_EDGE('',*,*,#3232,.F.);
#4650=ORIENTED_EDGE('',*,*,#3233,.T.);
#4651=ORIENTED_EDGE('',*,*,#3234,.T.);
#4652=ORIENTED_EDGE('',*,*,#3231,.F.);
#4653=ORIENTED_EDGE('',*,*,#3234,.F.);
#4654=ORIENTED_EDGE('',*,*,#3235,.T.);
#4655=ORIENTED_EDGE('',*,*,#3236,.T.);
#4656=ORIENTED_EDGE('',*,*,#3237,.F.);
#4657=ORIENTED_EDGE('',*,*,#3236,.F.);
#4658=ORIENTED_EDGE('',*,*,#3238,.T.);
#4659=ORIENTED_EDGE('',*,*,#3239,.T.);
#4660=ORIENTED_EDGE('',*,*,#3235,.F.);
#4661=ORIENTED_EDGE('',*,*,#3239,.F.);
#4662=ORIENTED_EDGE('',*,*,#3238,.F.);
#4663=ORIENTED_EDGE('',*,*,#3213,.T.);
#4664=ORIENTED_EDGE('',*,*,#3233,.F.);
#4665=ORIENTED_EDGE('',*,*,#3237,.T.);
#4666=ORIENTED_EDGE('',*,*,#3226,.F.);
#4667=ORIENTED_EDGE('',*,*,#3230,.T.);
#4668=ORIENTED_EDGE('',*,*,#3223,.T.);
#4669=ORIENTED_EDGE('',*,*,#3219,.F.);
#4670=ORIENTED_EDGE('',*,*,#3216,.T.);
#4671=ORIENTED_EDGE('',*,*,#3211,.F.);
#4819=PLANE('',#5595);
#4820=PLANE('',#5596);
#4821=PLANE('',#5597);
#4822=PLANE('',#5598);
#4823=PLANE('',#5628);
#4824=PLANE('',#5629);
#4825=PLANE('',#5630);
#4826=PLANE('',#5631);
#4827=PLANE('',#5668);
#4828=PLANE('',#5669);
#4829=PLANE('',#5670);
#4830=PLANE('',#5671);
#4831=PLANE('',#5672);
#4832=PLANE('',#5709);
#4833=PLANE('',#5710);
#4834=PLANE('',#5711);
#4835=PLANE('',#5712);
#4836=PLANE('',#5713);
#5054=ADVANCED_FACE('',(#692),#465,.F.);
#5055=ADVANCED_FACE('',(#693),#466,.F.);
#5056=ADVANCED_FACE('',(#694),#467,.F.);
#5057=ADVANCED_FACE('',(#695),#43,.F.);
#5058=ADVANCED_FACE('',(#696),#56,.T.);
#5059=ADVANCED_FACE('',(#697),#468,.T.);
#5060=ADVANCED_FACE('',(#698),#57,.T.);
#5061=ADVANCED_FACE('',(#699),#44,.F.);
#5062=ADVANCED_FACE('',(#700,#151),#4819,.F.);
#5063=ADVANCED_FACE('',(#701,#152),#4820,.F.);
#5064=ADVANCED_FACE('',(#702,#153),#4821,.F.);
#5065=ADVANCED_FACE('',(#703,#154),#4822,.F.);
#5066=ADVANCED_FACE('',(#704),#45,.T.);
#5067=ADVANCED_FACE('',(#705),#469,.T.);
#5068=ADVANCED_FACE('',(#706),#58,.F.);
#5069=ADVANCED_FACE('',(#707),#470,.T.);
#5070=ADVANCED_FACE('',(#708),#59,.F.);
#5071=ADVANCED_FACE('',(#709),#471,.T.);
#5072=ADVANCED_FACE('',(#710),#46,.T.);
#5073=ADVANCED_FACE('',(#711),#60,.T.);
#5074=ADVANCED_FACE('',(#712),#472,.F.);
#5075=ADVANCED_FACE('',(#713),#61,.T.);
#5076=ADVANCED_FACE('',(#714,#155),#4823,.F.);
#5077=ADVANCED_FACE('',(#715,#156),#4824,.F.);
#5078=ADVANCED_FACE('',(#716,#157),#4825,.F.);
#5079=ADVANCED_FACE('',(#717,#158),#4826,.F.);
#5080=ADVANCED_FACE('',(#718),#473,.F.);
#5081=ADVANCED_FACE('',(#719),#62,.T.);
#5082=ADVANCED_FACE('',(#720),#47,.T.);
#5083=ADVANCED_FACE('',(#721),#63,.F.);
#5084=ADVANCED_FACE('',(#722),#64,.F.);
#5085=ADVANCED_FACE('',(#723),#48,.F.);
#5086=ADVANCED_FACE('',(#724),#65,.F.);
#5087=ADVANCED_FACE('',(#725),#66,.T.);
#5088=ADVANCED_FACE('',(#726),#49,.T.);
#5089=ADVANCED_FACE('',(#727),#67,.T.);
#5090=ADVANCED_FACE('',(#728),#68,.T.);
#5091=ADVANCED_FACE('',(#729),#50,.F.);
#5092=ADVANCED_FACE('',(#730,#159),#4827,.F.);
#5093=ADVANCED_FACE('',(#731,#160),#4828,.F.);
#5094=ADVANCED_FACE('',(#732,#161),#4829,.T.);
#5095=ADVANCED_FACE('',(#733,#162),#4830,.T.);
#5096=ADVANCED_FACE('',(#734,#163),#4831,.T.);
#5097=ADVANCED_FACE('',(#735),#474,.F.);
#5098=ADVANCED_FACE('',(#736),#69,.T.);
#5099=ADVANCED_FACE('',(#737),#51,.T.);
#5100=ADVANCED_FACE('',(#738),#70,.F.);
#5101=ADVANCED_FACE('',(#739),#71,.F.);
#5102=ADVANCED_FACE('',(#740),#52,.F.);
#5103=ADVANCED_FACE('',(#741),#72,.F.);
#5104=ADVANCED_FACE('',(#742),#73,.T.);
#5105=ADVANCED_FACE('',(#743),#53,.T.);
#5106=ADVANCED_FACE('',(#744),#74,.T.);
#5107=ADVANCED_FACE('',(#745),#75,.T.);
#5108=ADVANCED_FACE('',(#746),#54,.F.);
#5109=ADVANCED_FACE('',(#747,#164),#4832,.F.);
#5110=ADVANCED_FACE('',(#748,#165),#4833,.F.);
#5111=ADVANCED_FACE('',(#749,#166),#4834,.T.);
#5112=ADVANCED_FACE('',(#750,#167),#4835,.T.);
#5113=ADVANCED_FACE('',(#751,#168),#4836,.T.);
#5120=CLOSED_SHELL('',(#5054,#5055,#5056,#5057,#5058,#5059,#5060,#5061,
#5062,#5063,#5064,#5065));
#5121=CLOSED_SHELL('',(#5066,#5067,#5068,#5069,#5070,#5071,#5072,#5073,
#5074,#5075,#5076,#5077,#5078,#5079));
#5122=CLOSED_SHELL('',(#5080,#5081,#5082,#5083,#5084,#5085,#5086,#5087,
#5088,#5089,#5090,#5091,#5092,#5093,#5094,#5095,#5096));
#5123=CLOSED_SHELL('',(#5097,#5098,#5099,#5100,#5101,#5102,#5103,#5104,
#5105,#5106,#5107,#5108,#5109,#5110,#5111,#5112,#5113));
#5571=AXIS2_PLACEMENT_3D('',#8527,#6923,#6924);
#5572=AXIS2_PLACEMENT_3D('',#8528,#6925,#6926);
#5573=AXIS2_PLACEMENT_3D('',#8530,#6927,#6928);
#5574=AXIS2_PLACEMENT_3D('',#8533,#6930,#6931);
#5575=AXIS2_PLACEMENT_3D('',#8534,#6932,#6933);
#5576=AXIS2_PLACEMENT_3D('',#8536,#6934,#6935);
#5577=AXIS2_PLACEMENT_3D('',#8539,#6937,#6938);
#5578=AXIS2_PLACEMENT_3D('',#8540,#6939,#6940);
#5579=AXIS2_PLACEMENT_3D('',#8543,#6941,#6942);
#5580=AXIS2_PLACEMENT_3D('',#8544,#6943,#6944);
#5581=AXIS2_PLACEMENT_3D('',#8547,#6946,#6947);
#5582=AXIS2_PLACEMENT_3D('',#8548,#6948,#6949);
#5583=AXIS2_PLACEMENT_3D('',#8551,#6951,#6952);
#5584=AXIS2_PLACEMENT_3D('',#8552,#6953,#6954);
#5585=AXIS2_PLACEMENT_3D('',#8554,#6955,#6956);
#5586=AXIS2_PLACEMENT_3D('',#8556,#6957,#6958);
#5587=AXIS2_PLACEMENT_3D('',#8557,#6959,#6960);
#5588=AXIS2_PLACEMENT_3D('',#8558,#6961,#6962);
#5589=AXIS2_PLACEMENT_3D('',#8560,#6963,#6964);
#5590=AXIS2_PLACEMENT_3D('',#8562,#6966,#6967);
#5591=AXIS2_PLACEMENT_3D('',#8564,#6968,#6969);
#5592=AXIS2_PLACEMENT_3D('',#8565,#6970,#6971);
#5593=AXIS2_PLACEMENT_3D('',#8566,#6972,#6973);
#5594=AXIS2_PLACEMENT_3D('',#8569,#6975,#6976);
#5595=AXIS2_PLACEMENT_3D('',#8570,#6977,#6978);
#5596=AXIS2_PLACEMENT_3D('',#8571,#6979,#6980);
#5597=AXIS2_PLACEMENT_3D('',#8572,#6981,#6982);
#5598=AXIS2_PLACEMENT_3D('',#8573,#6983,#6984);
#5599=AXIS2_PLACEMENT_3D('',#8574,#6985,#6986);
#5600=AXIS2_PLACEMENT_3D('',#8577,#6987,#6988);
#5601=AXIS2_PLACEMENT_3D('',#8580,#6990,#6991);
#5602=AXIS2_PLACEMENT_3D('',#8581,#6992,#6993);
#5603=AXIS2_PLACEMENT_3D('',#8582,#6994,#6995);
#5604=AXIS2_PLACEMENT_3D('',#8585,#6997,#6998);
#5605=AXIS2_PLACEMENT_3D('',#8586,#6999,#7000);
#5606=AXIS2_PLACEMENT_3D('',#8588,#7001,#7002);
#5607=AXIS2_PLACEMENT_3D('',#8589,#7003,#7004);
#5608=AXIS2_PLACEMENT_3D('',#8590,#7005,#7006);
#5609=AXIS2_PLACEMENT_3D('',#8592,#7007,#7008);
#5610=AXIS2_PLACEMENT_3D('',#8595,#7010,#7011);
#5611=AXIS2_PLACEMENT_3D('',#8596,#7012,#7013);
#5612=AXIS2_PLACEMENT_3D('',#8598,#7014,#7015);
#5613=AXIS2_PLACEMENT_3D('',#8600,#7016,#7017);
#5614=AXIS2_PLACEMENT_3D('',#8601,#7018,#7019);
#5615=AXIS2_PLACEMENT_3D('',#8602,#7020,#7021);
#5616=AXIS2_PLACEMENT_3D('',#8605,#7023,#7024);
#5617=AXIS2_PLACEMENT_3D('',#8606,#7025,#7026);
#5618=AXIS2_PLACEMENT_3D('',#8609,#7028,#7029);
#5619=AXIS2_PLACEMENT_3D('',#8610,#7030,#7031);
#5620=AXIS2_PLACEMENT_3D('',#8612,#7032,#7033);
#5621=AXIS2_PLACEMENT_3D('',#8614,#7034,#7035);
#5622=AXIS2_PLACEMENT_3D('',#8615,#7036,#7037);
#5623=AXIS2_PLACEMENT_3D('',#8616,#7038,#7039);
#5624=AXIS2_PLACEMENT_3D('',#8619,#7041,#7042);
#5625=AXIS2_PLACEMENT_3D('',#8620,#7043,#7044);
#5626=AXIS2_PLACEMENT_3D('',#8622,#7045,#7046);
#5627=AXIS2_PLACEMENT_3D('',#8623,#7047,#7048);
#5628=AXIS2_PLACEMENT_3D('',#8624,#7049,#7050);
#5629=AXIS2_PLACEMENT_3D('',#8625,#7051,#7052);
#5630=AXIS2_PLACEMENT_3D('',#8626,#7053,#7054);
#5631=AXIS2_PLACEMENT_3D('',#8627,#7055,#7056);
#5632=AXIS2_PLACEMENT_3D('',#8628,#7057,#7058);
#5633=AXIS2_PLACEMENT_3D('',#8630,#7059,#7060);
#5634=AXIS2_PLACEMENT_3D('',#8633,#7062,#7063);
#5635=AXIS2_PLACEMENT_3D('',#8634,#7064,#7065);
#5636=AXIS2_PLACEMENT_3D('',#8636,#7066,#7067);
#5637=AXIS2_PLACEMENT_3D('',#8638,#7068,#7069);
#5638=AXIS2_PLACEMENT_3D('',#8639,#7070,#7071);
#5639=AXIS2_PLACEMENT_3D('',#8640,#7072,#7073);
#5640=AXIS2_PLACEMENT_3D('',#8642,#7074,#7075);
#5641=AXIS2_PLACEMENT_3D('',#8644,#7077,#7078);
#5642=AXIS2_PLACEMENT_3D('',#8646,#7079,#7080);
#5643=AXIS2_PLACEMENT_3D('',#8647,#7081,#7082);
#5644=AXIS2_PLACEMENT_3D('',#8648,#7083,#7084);
#5645=AXIS2_PLACEMENT_3D('',#8650,#7085,#7086);
#5646=AXIS2_PLACEMENT_3D('',#8652,#7087,#7088);
#5647=AXIS2_PLACEMENT_3D('',#8653,#7089,#7090);
#5648=AXIS2_PLACEMENT_3D('',#8654,#7091,#7092);
#5649=AXIS2_PLACEMENT_3D('',#8656,#7093,#7094);
#5650=AXIS2_PLACEMENT_3D('',#8658,#7096,#7097);
#5651=AXIS2_PLACEMENT_3D('',#8660,#7098,#7099);
#5652=AXIS2_PLACEMENT_3D('',#8661,#7100,#7101);
#5653=AXIS2_PLACEMENT_3D('',#8662,#7102,#7103);
#5654=AXIS2_PLACEMENT_3D('',#8664,#7104,#7105);
#5655=AXIS2_PLACEMENT_3D('',#8666,#7106,#7107);
#5656=AXIS2_PLACEMENT_3D('',#8667,#7108,#7109);
#5657=AXIS2_PLACEMENT_3D('',#8668,#7110,#7111);
#5658=AXIS2_PLACEMENT_3D('',#8670,#7112,#7113);
#5659=AXIS2_PLACEMENT_3D('',#8672,#7115,#7116);
#5660=AXIS2_PLACEMENT_3D('',#8674,#7117,#7118);
#5661=AXIS2_PLACEMENT_3D('',#8675,#7119,#7120);
#5662=AXIS2_PLACEMENT_3D('',#8676,#7121,#7122);
#5663=AXIS2_PLACEMENT_3D('',#8678,#7123,#7124);
#5664=AXIS2_PLACEMENT_3D('',#8680,#7125,#7126);
#5665=AXIS2_PLACEMENT_3D('',#8681,#7127,#7128);
#5666=AXIS2_PLACEMENT_3D('',#8682,#7129,#7130);
#5667=AXIS2_PLACEMENT_3D('',#8684,#7131,#7132);
#5668=AXIS2_PLACEMENT_3D('',#8686,#7134,#7135);
#5669=AXIS2_PLACEMENT_3D('',#8687,#7136,#7137);
#5670=AXIS2_PLACEMENT_3D('',#8688,#7138,#7139);
#5671=AXIS2_PLACEMENT_3D('',#8689,#7140,#7141);
#5672=AXIS2_PLACEMENT_3D('',#8690,#7142,#7143);
#5673=AXIS2_PLACEMENT_3D('',#8691,#7144,#7145);
#5674=AXIS2_PLACEMENT_3D('',#8693,#7146,#7147);
#5675=AXIS2_PLACEMENT_3D('',#8696,#7149,#7150);
#5676=AXIS2_PLACEMENT_3D('',#8697,#7151,#7152);
#5677=AXIS2_PLACEMENT_3D('',#8699,#7153,#7154);
#5678=AXIS2_PLACEMENT_3D('',#8701,#7155,#7156);
#5679=AXIS2_PLACEMENT_3D('',#8702,#7157,#7158);
#5680=AXIS2_PLACEMENT_3D('',#8703,#7159,#7160);
#5681=AXIS2_PLACEMENT_3D('',#8705,#7161,#7162);
#5682=AXIS2_PLACEMENT_3D('',#8707,#7164,#7165);
#5683=AXIS2_PLACEMENT_3D('',#8709,#7166,#7167);
#5684=AXIS2_PLACEMENT_3D('',#8710,#7168,#7169);
#5685=AXIS2_PLACEMENT_3D('',#8711,#7170,#7171);
#5686=AXIS2_PLACEMENT_3D('',#8713,#7172,#7173);
#5687=AXIS2_PLACEMENT_3D('',#8715,#7174,#7175);
#5688=AXIS2_PLACEMENT_3D('',#8716,#7176,#7177);
#5689=AXIS2_PLACEMENT_3D('',#8717,#7178,#7179);
#5690=AXIS2_PLACEMENT_3D('',#8719,#7180,#7181);
#5691=AXIS2_PLACEMENT_3D('',#8721,#7183,#7184);
#5692=AXIS2_PLACEMENT_3D('',#8723,#7185,#7186);
#5693=AXIS2_PLACEMENT_3D('',#8724,#7187,#7188);
#5694=AXIS2_PLACEMENT_3D('',#8725,#7189,#7190);
#5695=AXIS2_PLACEMENT_3D('',#8727,#7191,#7192);
#5696=AXIS2_PLACEMENT_3D('',#8729,#7193,#7194);
#5697=AXIS2_PLACEMENT_3D('',#8730,#7195,#7196);
#5698=AXIS2_PLACEMENT_3D('',#8731,#7197,#7198);
#5699=AXIS2_PLACEMENT_3D('',#8733,#7199,#7200);
#5700=AXIS2_PLACEMENT_3D('',#8735,#7202,#7203);
#5701=AXIS2_PLACEMENT_3D('',#8737,#7204,#7205);
#5702=AXIS2_PLACEMENT_3D('',#8738,#7206,#7207);
#5703=AXIS2_PLACEMENT_3D('',#8739,#7208,#7209);
#5704=AXIS2_PLACEMENT_3D('',#8741,#7210,#7211);
#5705=AXIS2_PLACEMENT_3D('',#8743,#7212,#7213);
#5706=AXIS2_PLACEMENT_3D('',#8744,#7214,#7215);
#5707=AXIS2_PLACEMENT_3D('',#8745,#7216,#7217);
#5708=AXIS2_PLACEMENT_3D('',#8747,#7218,#7219);
#5709=AXIS2_PLACEMENT_3D('',#8749,#7221,#7222);
#5710=AXIS2_PLACEMENT_3D('',#8750,#7223,#7224);
#5711=AXIS2_PLACEMENT_3D('',#8751,#7225,#7226);
#5712=AXIS2_PLACEMENT_3D('',#8752,#7227,#7228);
#5713=AXIS2_PLACEMENT_3D('',#8753,#7229,#7230);
#6923=DIRECTION('axis',(0.,0.,1.));
#6924=DIRECTION('refdir',(1.,0.,0.));
#6925=DIRECTION('center_axis',(-1.,-1.83697019872103E-16,0.));
#6926=DIRECTION('ref_axis',(1.83697019872103E-16,-1.,0.));
#6927=DIRECTION('center_axis',(-1.,-1.83697019872103E-16,0.));
#6928=DIRECTION('ref_axis',(1.83697019872103E-16,-1.,0.));
#6929=DIRECTION('',(-1.,-1.83697019872103E-16,0.));
#6930=DIRECTION('center_axis',(-1.,-1.83697019872103E-16,0.));
#6931=DIRECTION('ref_axis',(1.83697019872103E-16,-1.,0.));
#6932=DIRECTION('center_axis',(-1.,-1.83697019872103E-16,0.));
#6933=DIRECTION('ref_axis',(1.83697019872103E-16,-1.,0.));
#6934=DIRECTION('center_axis',(-1.,-1.83697019872103E-16,0.));
#6935=DIRECTION('ref_axis',(1.83697019872103E-16,-1.,0.));
#6936=DIRECTION('',(-1.,-1.83697019872103E-16,0.));
#6937=DIRECTION('center_axis',(-1.,-1.83697019872103E-16,0.));
#6938=DIRECTION('ref_axis',(1.83697019872103E-16,-1.,0.));
#6939=DIRECTION('center_axis',(-1.,-1.83697019872103E-16,0.));
#6940=DIRECTION('ref_axis',(1.83697019872103E-16,-1.,0.));
#6941=DIRECTION('center_axis',(-1.,-1.83697019872103E-16,0.));
#6942=DIRECTION('ref_axis',(1.83697019872103E-16,-1.,0.));
#6943=DIRECTION('center_axis',(-1.,-1.83697019872103E-16,0.));
#6944=DIRECTION('ref_axis',(1.83697019872103E-16,-1.,0.));
#6945=DIRECTION('',(-1.,-1.83697019872103E-16,0.));
#6946=DIRECTION('center_axis',(-1.,-1.83697019872103E-16,0.));
#6947=DIRECTION('ref_axis',(1.83697019872103E-16,-1.,0.));
#6948=DIRECTION('center_axis',(1.,1.83697019872103E-16,0.));
#6949=DIRECTION('ref_axis',(-1.83697019872103E-16,1.,0.));
#6950=DIRECTION('',(0.707106781186551,-0.707106781186544,-8.6595605623549E-17));
#6951=DIRECTION('center_axis',(-1.,-1.83697019872103E-16,0.));
#6952=DIRECTION('ref_axis',(1.83697019872103E-16,-1.,0.));
#6953=DIRECTION('center_axis',(-1.,-1.83697019872103E-16,0.));
#6954=DIRECTION('ref_axis',(1.85037170770859E-16,-1.,0.));
#6955=DIRECTION('center_axis',(-1.,-1.83697019872103E-16,0.));
#6956=DIRECTION('ref_axis',(1.83697019872103E-16,-1.,0.));
#6957=DIRECTION('center_axis',(2.24963967399279E-32,-1.22464679914735E-16,
-1.));
#6958=DIRECTION('ref_axis',(-1.85037170770859E-16,1.,-1.22464679914735E-16));
#6959=DIRECTION('center_axis',(-1.,-1.83697019872103E-16,0.));
#6960=DIRECTION('ref_axis',(1.83697019872103E-16,-1.,0.));
#6961=DIRECTION('center_axis',(-1.,-1.83697019872103E-16,0.));
#6962=DIRECTION('ref_axis',(1.83697019872103E-16,-1.,0.));
#6963=DIRECTION('center_axis',(-1.,-1.83697019872103E-16,0.));
#6964=DIRECTION('ref_axis',(1.83697019872103E-16,-1.,0.));
#6965=DIRECTION('',(1.,1.83697019872103E-16,0.));
#6966=DIRECTION('center_axis',(-1.,-1.83697019872103E-16,0.));
#6967=DIRECTION('ref_axis',(1.85037170770859E-16,-1.,0.));
#6968=DIRECTION('center_axis',(-1.,-1.83697019872103E-16,0.));
#6969=DIRECTION('ref_axis',(1.83697019872103E-16,-1.,0.));
#6970=DIRECTION('center_axis',(2.24963967399279E-32,-1.22464679914735E-16,
-1.));
#6971=DIRECTION('ref_axis',(-1.85037170770859E-16,1.,-1.22464679914735E-16));
#6972=DIRECTION('center_axis',(-1.,-1.83697019872103E-16,0.));
#6973=DIRECTION('ref_axis',(1.83697019872103E-16,-1.,0.));
#6974=DIRECTION('',(-0.707106781186551,0.707106781186544,-8.6595605623549E-17));
#6975=DIRECTION('center_axis',(-1.,-1.83697019872103E-16,0.));
#6976=DIRECTION('ref_axis',(1.83697019872103E-16,-1.,0.));
#6977=DIRECTION('center_axis',(1.,1.83697019872103E-16,0.));
#6978=DIRECTION('ref_axis',(-1.83697019872103E-16,1.,0.));
#6979=DIRECTION('center_axis',(-1.,-1.83697019872103E-16,0.));
#6980=DIRECTION('ref_axis',(1.83697019872103E-16,-1.,0.));
#6981=DIRECTION('center_axis',(1.,1.83697019872103E-16,0.));
#6982=DIRECTION('ref_axis',(-1.83697019872103E-16,1.,0.));
#6983=DIRECTION('center_axis',(-1.,-1.83697019872103E-16,0.));
#6984=DIRECTION('ref_axis',(1.83697019872103E-16,-1.,0.));
#6985=DIRECTION('center_axis',(1.,1.83697019872103E-16,0.));
#6986=DIRECTION('ref_axis',(-1.83697019872103E-16,1.,0.));
#6987=DIRECTION('center_axis',(-1.,-1.83697019872103E-16,0.));
#6988=DIRECTION('ref_axis',(1.83697019872103E-16,-1.,0.));
#6989=DIRECTION('',(-0.707106781186548,0.707106781186547,8.65956056235493E-17));
#6990=DIRECTION('center_axis',(-1.,-1.83697019872103E-16,0.));
#6991=DIRECTION('ref_axis',(1.83697019872103E-16,-1.,0.));
#6992=DIRECTION('center_axis',(-1.,-1.83697019872103E-16,0.));
#6993=DIRECTION('ref_axis',(1.83697019872103E-16,-1.,0.));
#6994=DIRECTION('center_axis',(-1.,-1.83697019872103E-16,0.));
#6995=DIRECTION('ref_axis',(1.83697019872103E-16,-1.,0.));
#6996=DIRECTION('',(1.,1.83697019872103E-16,0.));
#6997=DIRECTION('center_axis',(-1.,-1.83697019872103E-16,0.));
#6998=DIRECTION('ref_axis',(1.83697019872103E-16,-1.,0.));
#6999=DIRECTION('center_axis',(-1.,-1.83697019872103E-16,0.));
#7000=DIRECTION('ref_axis',(1.96129949112834E-16,-1.,0.));
#7001=DIRECTION('center_axis',(-2.24963967399279E-32,1.22464679914735E-16,
1.));
#7002=DIRECTION('ref_axis',(-1.63441624260695E-16,1.,-1.22464679914735E-16));
#7003=DIRECTION('center_axis',(-1.,-1.83697019872103E-16,0.));
#7004=DIRECTION('ref_axis',(1.83697019872103E-16,-1.,0.));
#7005=DIRECTION('center_axis',(-1.,-1.83697019872103E-16,0.));
#7006=DIRECTION('ref_axis',(1.83697019872103E-16,-1.,0.));
#7007=DIRECTION('center_axis',(-1.,-1.83697019872103E-16,0.));
#7008=DIRECTION('ref_axis',(1.83697019872103E-16,-1.,0.));
#7009=DIRECTION('',(1.,1.83697019872103E-16,0.));
#7010=DIRECTION('center_axis',(-1.,-1.83697019872103E-16,0.));
#7011=DIRECTION('ref_axis',(1.83697019872103E-16,-1.,0.));
#7012=DIRECTION('center_axis',(-1.,-1.83697019872103E-16,0.));
#7013=DIRECTION('ref_axis',(1.96129949112834E-16,-1.,0.));
#7014=DIRECTION('center_axis',(-1.,-1.83697019872103E-16,0.));
#7015=DIRECTION('ref_axis',(1.83697019872103E-16,-1.,0.));
#7016=DIRECTION('center_axis',(-2.24963967399279E-32,1.22464679914735E-16,
1.));
#7017=DIRECTION('ref_axis',(-1.63441624260695E-16,1.,-1.22464679914735E-16));
#7018=DIRECTION('center_axis',(-1.,-1.83697019872103E-16,0.));
#7019=DIRECTION('ref_axis',(1.83697019872103E-16,-1.,0.));
#7020=DIRECTION('center_axis',(-1.,-1.83697019872103E-16,0.));
#7021=DIRECTION('ref_axis',(1.83697019872103E-16,-1.,0.));
#7022=DIRECTION('',(1.,1.83697019872103E-16,0.));
#7023=DIRECTION('center_axis',(-1.,-1.83697019872103E-16,0.));
#7024=DIRECTION('ref_axis',(1.83697019872103E-16,-1.,0.));
#7025=DIRECTION('center_axis',(-1.,-1.83697019872103E-16,0.));
#7026=DIRECTION('ref_axis',(1.83697019872103E-16,-1.,0.));
#7027=DIRECTION('',(0.707106781186548,-0.707106781186547,8.65956056235493E-17));
#7028=DIRECTION('center_axis',(-1.,-1.83697019872103E-16,0.));
#7029=DIRECTION('ref_axis',(1.83697019872103E-16,-1.,0.));
#7030=DIRECTION('center_axis',(-1.,-1.83697019872103E-16,0.));
#7031=DIRECTION('ref_axis',(1.85037170770859E-16,-1.,0.));
#7032=DIRECTION('center_axis',(-1.,-1.83697019872103E-16,0.));
#7033=DIRECTION('ref_axis',(1.83697019872103E-16,-1.,0.));
#7034=DIRECTION('center_axis',(2.24963967399279E-32,-1.22464679914735E-16,
-1.));
#7035=DIRECTION('ref_axis',(-2.31296463463574E-16,1.,-1.22464679914735E-16));
#7036=DIRECTION('center_axis',(-1.,-1.83697019872103E-16,0.));
#7037=DIRECTION('ref_axis',(1.83697019872103E-16,-1.,0.));
#7038=DIRECTION('center_axis',(-1.,-1.83697019872103E-16,0.));
#7039=DIRECTION('ref_axis',(1.83697019872103E-16,-1.,0.));
#7040=DIRECTION('',(-1.,-1.83697019872103E-16,0.));
#7041=DIRECTION('center_axis',(-1.,-1.83697019872103E-16,0.));
#7042=DIRECTION('ref_axis',(1.83697019872103E-16,-1.,0.));
#7043=DIRECTION('center_axis',(-1.,-1.83697019872103E-16,0.));
#7044=DIRECTION('ref_axis',(1.85037170770859E-16,-1.,0.));
#7045=DIRECTION('center_axis',(2.24963967399279E-32,-1.22464679914735E-16,
-1.));
#7046=DIRECTION('ref_axis',(-2.31296463463574E-16,1.,-1.22464679914735E-16));
#7047=DIRECTION('center_axis',(-1.,-1.83697019872103E-16,0.));
#7048=DIRECTION('ref_axis',(1.83697019872103E-16,-1.,0.));
#7049=DIRECTION('center_axis',(-1.,-1.83697019872103E-16,0.));
#7050=DIRECTION('ref_axis',(1.83697019872103E-16,-1.,0.));
#7051=DIRECTION('center_axis',(-1.,-1.83697019872103E-16,0.));
#7052=DIRECTION('ref_axis',(1.83697019872103E-16,-1.,0.));
#7053=DIRECTION('center_axis',(1.,1.83697019872103E-16,0.));
#7054=DIRECTION('ref_axis',(-1.83697019872103E-16,1.,0.));
#7055=DIRECTION('center_axis',(1.,1.83697019872103E-16,0.));
#7056=DIRECTION('ref_axis',(-1.83697019872103E-16,1.,0.));
#7057=DIRECTION('center_axis',(-1.,-1.83697019872103E-16,0.));
#7058=DIRECTION('ref_axis',(1.83697019872103E-16,-1.,0.));
#7059=DIRECTION('center_axis',(-1.,-1.83697019872103E-16,0.));
#7060=DIRECTION('ref_axis',(1.83697019872103E-16,-1.,0.));
#7061=DIRECTION('',(-1.,-1.83697019872103E-16,0.));
#7062=DIRECTION('center_axis',(-1.,-1.83697019872103E-16,0.));
#7063=DIRECTION('ref_axis',(1.83697019872103E-16,-1.,0.));
#7064=DIRECTION('center_axis',(-1.,-1.83697019872103E-16,0.));
#7065=DIRECTION('ref_axis',(1.57361694361665E-16,-1.,0.));
#7066=DIRECTION('center_axis',(-1.,-1.83697019872103E-16,0.));
#7067=DIRECTION('ref_axis',(1.83697019872103E-16,-1.,0.));
#7068=DIRECTION('center_axis',(2.24963967399279E-32,-1.22464679914735E-16,
-1.));
#7069=DIRECTION('ref_axis',(-1.96702117952081E-16,1.,-1.22464679914735E-16));
#7070=DIRECTION('center_axis',(-1.,-1.83697019872103E-16,0.));
#7071=DIRECTION('ref_axis',(1.83697019872103E-16,-1.,0.));
#7072=DIRECTION('center_axis',(-1.,-1.83697019872103E-16,0.));
#7073=DIRECTION('ref_axis',(1.83697019872103E-16,-1.,0.));
#7074=DIRECTION('center_axis',(-1.,-1.83697019872103E-16,0.));
#7075=DIRECTION('ref_axis',(1.83697019872103E-16,-1.,0.));
#7076=DIRECTION('',(0.866025403784443,-0.499999999999992,6.12323399573667E-17));
#7077=DIRECTION('center_axis',(-1.,-1.83697019872103E-16,0.));
#7078=DIRECTION('ref_axis',(2.01689087919369E-16,-1.,0.));
#7079=DIRECTION('center_axis',(-1.,-1.83697019872103E-16,0.));
#7080=DIRECTION('ref_axis',(1.83697019872103E-16,-1.,0.));
#7081=DIRECTION('center_axis',(-2.24963967399279E-32,1.22464679914735E-16,
1.));
#7082=DIRECTION('ref_axis',(-1.89083519924408E-16,1.,-1.22464679914735E-16));
#7083=DIRECTION('center_axis',(-1.,-1.83697019872103E-16,0.));
#7084=DIRECTION('ref_axis',(1.88974131851091E-16,-1.,0.));
#7085=DIRECTION('center_axis',(-1.,-1.83697019872103E-16,0.));
#7086=DIRECTION('ref_axis',(1.83697019872103E-16,-1.,0.));
#7087=DIRECTION('center_axis',(-2.24963967399279E-32,1.22464679914735E-16,
1.));
#7088=DIRECTION('ref_axis',(-1.77163248610397E-16,1.,-1.22464679914735E-16));
#7089=DIRECTION('center_axis',(-1.,-1.83697019872103E-16,0.));
#7090=DIRECTION('ref_axis',(1.83697019872103E-16,-1.,0.));
#7091=DIRECTION('center_axis',(-1.,-1.83697019872103E-16,0.));
#7092=DIRECTION('ref_axis',(1.83697019872103E-16,-1.,0.));
#7093=DIRECTION('center_axis',(-1.,-1.83697019872103E-16,0.));
#7094=DIRECTION('ref_axis',(1.83697019872103E-16,-1.,0.));
#7095=DIRECTION('',(-0.500000000000007,0.866025403784435,-1.0605752387249E-16));
#7096=DIRECTION('center_axis',(-1.,-1.83697019872103E-16,0.));
#7097=DIRECTION('ref_axis',(1.91801449774277E-16,-1.,0.));
#7098=DIRECTION('center_axis',(-1.,-1.83697019872103E-16,0.));
#7099=DIRECTION('ref_axis',(1.83697019872103E-16,-1.,0.));
#7100=DIRECTION('center_axis',(-2.24963967399279E-32,1.22464679914735E-16,
1.));
#7101=DIRECTION('ref_axis',(-1.79813859163385E-16,1.,-1.22464679914735E-16));
#7102=DIRECTION('center_axis',(-1.,-1.83697019872103E-16,0.));
#7103=DIRECTION('ref_axis',(1.87747066251861E-16,-1.,0.));
#7104=DIRECTION('center_axis',(-1.,-1.83697019872103E-16,0.));
#7105=DIRECTION('ref_axis',(1.83697019872103E-16,-1.,0.));
#7106=DIRECTION('center_axis',(2.24963967399279E-32,-1.22464679914735E-16,
-1.));
#7107=DIRECTION('ref_axis',(-1.7601287461112E-16,1.,-1.22464679914735E-16));
#7108=DIRECTION('center_axis',(-1.,-1.83697019872103E-16,0.));
#7109=DIRECTION('ref_axis',(1.83697019872103E-16,-1.,0.));
#7110=DIRECTION('center_axis',(-1.,-1.83697019872103E-16,0.));
#7111=DIRECTION('ref_axis',(1.83697019872103E-16,-1.,0.));
#7112=DIRECTION('center_axis',(-1.,-1.83697019872103E-16,0.));
#7113=DIRECTION('ref_axis',(1.83697019872103E-16,-1.,0.));
#7114=DIRECTION('',(0.500000000000007,-0.866025403784435,1.0605752387249E-16));
#7115=DIRECTION('center_axis',(-1.,-1.83697019872103E-16,0.));
#7116=DIRECTION('ref_axis',(1.85037170770859E-16,-1.,0.));
#7117=DIRECTION('center_axis',(-1.,-1.83697019872103E-16,0.));
#7118=DIRECTION('ref_axis',(1.83697019872103E-16,-1.,0.));
#7119=DIRECTION('center_axis',(2.24963967399279E-32,-1.22464679914735E-16,
-1.));
#7120=DIRECTION('ref_axis',(-1.73472347597681E-16,1.,-1.22464679914735E-16));
#7121=DIRECTION('center_axis',(-1.,-1.83697019872103E-16,0.));
#7122=DIRECTION('ref_axis',(1.97210791246963E-16,-1.,0.));
#7123=DIRECTION('center_axis',(-1.,-1.83697019872103E-16,0.));
#7124=DIRECTION('ref_axis',(1.83697019872103E-16,-1.,0.));
#7125=DIRECTION('center_axis',(2.24963967399279E-32,-1.22464679914735E-16,
-1.));
#7126=DIRECTION('ref_axis',(-1.84885116794028E-16,1.,-1.22464679914735E-16));
#7127=DIRECTION('center_axis',(-1.,-1.83697019872103E-16,0.));
#7128=DIRECTION('ref_axis',(1.83697019872103E-16,-1.,0.));
#7129=DIRECTION('center_axis',(-1.,-1.83697019872103E-16,0.));
#7130=DIRECTION('ref_axis',(1.83697019872103E-16,-1.,0.));
#7131=DIRECTION('center_axis',(-1.,-1.83697019872103E-16,0.));
#7132=DIRECTION('ref_axis',(1.83697019872103E-16,-1.,0.));
#7133=DIRECTION('',(-0.866025403784443,0.499999999999992,-6.12323399573667E-17));
#7134=DIRECTION('center_axis',(1.,1.83697019872103E-16,0.));
#7135=DIRECTION('ref_axis',(-1.83697019872103E-16,1.,0.));
#7136=DIRECTION('center_axis',(1.,1.83697019872103E-16,0.));
#7137=DIRECTION('ref_axis',(-1.83697019872103E-16,1.,0.));
#7138=DIRECTION('center_axis',(-1.,-1.83697019872103E-16,0.));
#7139=DIRECTION('ref_axis',(1.83697019872103E-16,-1.,0.));
#7140=DIRECTION('center_axis',(1.,1.83697019872103E-16,0.));
#7141=DIRECTION('ref_axis',(-1.83697019872103E-16,1.,0.));
#7142=DIRECTION('center_axis',(1.,1.83697019872103E-16,0.));
#7143=DIRECTION('ref_axis',(-1.83697019872103E-16,1.,0.));
#7144=DIRECTION('center_axis',(1.,-1.83697019872103E-16,0.));
#7145=DIRECTION('ref_axis',(-1.83697019872103E-16,-1.,0.));
#7146=DIRECTION('center_axis',(-1.,1.83697019872103E-16,0.));
#7147=DIRECTION('ref_axis',(-1.83697019872103E-16,-1.,0.));
#7148=DIRECTION('',(1.,-1.83697019872103E-16,0.));
#7149=DIRECTION('center_axis',(-1.,1.83697019872103E-16,0.));
#7150=DIRECTION('ref_axis',(-1.83697019872103E-16,-1.,0.));
#7151=DIRECTION('center_axis',(1.,-1.83697019872103E-16,0.));
#7152=DIRECTION('ref_axis',(-1.57361694361665E-16,-1.,0.));
#7153=DIRECTION('center_axis',(-1.,1.83697019872103E-16,0.));
#7154=DIRECTION('ref_axis',(-1.83697019872103E-16,-1.,0.));
#7155=DIRECTION('center_axis',(-2.24963967399279E-32,-1.22464679914735E-16,
1.));
#7156=DIRECTION('ref_axis',(1.96702117952081E-16,1.,1.22464679914735E-16));
#7157=DIRECTION('center_axis',(-1.,1.83697019872103E-16,0.));
#7158=DIRECTION('ref_axis',(-1.83697019872103E-16,-1.,0.));
#7159=DIRECTION('center_axis',(1.,-1.83697019872103E-16,0.));
#7160=DIRECTION('ref_axis',(-1.83697019872103E-16,-1.,0.));
#7161=DIRECTION('center_axis',(-1.,1.83697019872103E-16,0.));
#7162=DIRECTION('ref_axis',(-1.83697019872103E-16,-1.,0.));
#7163=DIRECTION('',(-0.866025403784443,-0.499999999999992,-6.12323399573667E-17));
#7164=DIRECTION('center_axis',(1.,-1.83697019872103E-16,0.));
#7165=DIRECTION('ref_axis',(-2.01689087919369E-16,-1.,0.));
#7166=DIRECTION('center_axis',(-1.,1.83697019872103E-16,0.));
#7167=DIRECTION('ref_axis',(-1.83697019872103E-16,-1.,0.));
#7168=DIRECTION('center_axis',(2.24963967399279E-32,1.22464679914735E-16,
-1.));
#7169=DIRECTION('ref_axis',(1.89083519924408E-16,1.,1.22464679914735E-16));
#7170=DIRECTION('center_axis',(1.,-1.83697019872103E-16,0.));
#7171=DIRECTION('ref_axis',(-1.88974131851091E-16,-1.,0.));
#7172=DIRECTION('center_axis',(-1.,1.83697019872103E-16,0.));
#7173=DIRECTION('ref_axis',(-1.83697019872103E-16,-1.,0.));
#7174=DIRECTION('center_axis',(2.24963967399279E-32,1.22464679914735E-16,
-1.));
#7175=DIRECTION('ref_axis',(1.77163248610397E-16,1.,1.22464679914735E-16));
#7176=DIRECTION('center_axis',(-1.,1.83697019872103E-16,0.));
#7177=DIRECTION('ref_axis',(-1.83697019872103E-16,-1.,0.));
#7178=DIRECTION('center_axis',(1.,-1.83697019872103E-16,0.));
#7179=DIRECTION('ref_axis',(-1.83697019872103E-16,-1.,0.));
#7180=DIRECTION('center_axis',(-1.,1.83697019872103E-16,0.));
#7181=DIRECTION('ref_axis',(-1.83697019872103E-16,-1.,0.));
#7182=DIRECTION('',(0.500000000000007,0.866025403784435,1.0605752387249E-16));
#7183=DIRECTION('center_axis',(1.,-1.83697019872103E-16,0.));
#7184=DIRECTION('ref_axis',(-1.91801449774277E-16,-1.,0.));
#7185=DIRECTION('center_axis',(-1.,1.83697019872103E-16,0.));
#7186=DIRECTION('ref_axis',(-1.83697019872103E-16,-1.,0.));
#7187=DIRECTION('center_axis',(2.24963967399279E-32,1.22464679914735E-16,
-1.));
#7188=DIRECTION('ref_axis',(1.79813859163385E-16,1.,1.22464679914735E-16));
#7189=DIRECTION('center_axis',(1.,-1.83697019872103E-16,0.));
#7190=DIRECTION('ref_axis',(-1.87747066251861E-16,-1.,0.));
#7191=DIRECTION('center_axis',(-1.,1.83697019872103E-16,0.));
#7192=DIRECTION('ref_axis',(-1.83697019872103E-16,-1.,0.));
#7193=DIRECTION('center_axis',(-2.24963967399279E-32,-1.22464679914735E-16,
1.));
#7194=DIRECTION('ref_axis',(1.7601287461112E-16,1.,1.22464679914735E-16));
#7195=DIRECTION('center_axis',(-1.,1.83697019872103E-16,0.));
#7196=DIRECTION('ref_axis',(-1.83697019872103E-16,-1.,0.));
#7197=DIRECTION('center_axis',(1.,-1.83697019872103E-16,0.));
#7198=DIRECTION('ref_axis',(-1.83697019872103E-16,-1.,0.));
#7199=DIRECTION('center_axis',(-1.,1.83697019872103E-16,0.));
#7200=DIRECTION('ref_axis',(-1.83697019872103E-16,-1.,0.));
#7201=DIRECTION('',(-0.500000000000007,-0.866025403784435,-1.0605752387249E-16));
#7202=DIRECTION('center_axis',(1.,-1.83697019872103E-16,0.));
#7203=DIRECTION('ref_axis',(-1.85037170770859E-16,-1.,0.));
#7204=DIRECTION('center_axis',(-1.,1.83697019872103E-16,0.));
#7205=DIRECTION('ref_axis',(-1.83697019872103E-16,-1.,0.));
#7206=DIRECTION('center_axis',(-2.24963967399279E-32,-1.22464679914735E-16,
1.));
#7207=DIRECTION('ref_axis',(1.73472347597681E-16,1.,1.22464679914735E-16));
#7208=DIRECTION('center_axis',(1.,-1.83697019872103E-16,0.));
#7209=DIRECTION('ref_axis',(-1.97210791246963E-16,-1.,0.));
#7210=DIRECTION('center_axis',(-1.,1.83697019872103E-16,0.));
#7211=DIRECTION('ref_axis',(-1.83697019872103E-16,-1.,0.));
#7212=DIRECTION('center_axis',(-2.24963967399279E-32,-1.22464679914735E-16,
1.));
#7213=DIRECTION('ref_axis',(1.84885116794028E-16,1.,1.22464679914735E-16));
#7214=DIRECTION('center_axis',(-1.,1.83697019872103E-16,0.));
#7215=DIRECTION('ref_axis',(-1.83697019872103E-16,-1.,0.));
#7216=DIRECTION('center_axis',(1.,-1.83697019872103E-16,0.));
#7217=DIRECTION('ref_axis',(-1.83697019872103E-16,-1.,0.));
#7218=DIRECTION('center_axis',(-1.,1.83697019872103E-16,0.));
#7219=DIRECTION('ref_axis',(-1.83697019872103E-16,-1.,0.));
#7220=DIRECTION('',(0.866025403784443,0.499999999999992,6.12323399573667E-17));
#7221=DIRECTION('center_axis',(-1.,1.83697019872103E-16,0.));
#7222=DIRECTION('ref_axis',(1.83697019872103E-16,1.,0.));
#7223=DIRECTION('center_axis',(-1.,1.83697019872103E-16,0.));
#7224=DIRECTION('ref_axis',(1.83697019872103E-16,1.,0.));
#7225=DIRECTION('center_axis',(1.,-1.83697019872103E-16,0.));
#7226=DIRECTION('ref_axis',(-1.83697019872103E-16,-1.,0.));
#7227=DIRECTION('center_axis',(-1.,1.83697019872103E-16,0.));
#7228=DIRECTION('ref_axis',(1.83697019872103E-16,1.,0.));
#7229=DIRECTION('center_axis',(-1.,1.83697019872103E-16,0.));
#7230=DIRECTION('ref_axis',(1.83697019872103E-16,1.,0.));
#8527=CARTESIAN_POINT('',(0.,0.,0.));
#8528=CARTESIAN_POINT('Origin',(-1.8,0.,0.));
#8529=CARTESIAN_POINT('',(-1.7,4.8,-5.8783046359073E-16));
#8530=CARTESIAN_POINT('Origin',(-1.7,1.83697019872105E-17,0.));
#8531=CARTESIAN_POINT('',(-1.955,4.8,-5.8783046359073E-16));
#8532=CARTESIAN_POINT('',(-1.8,4.8,-5.87830463590729E-16));
#8533=CARTESIAN_POINT('Origin',(-1.955,-2.84730380801758E-17,0.));
#8534=CARTESIAN_POINT('Origin',(-1.8,0.,0.));
#8535=CARTESIAN_POINT('',(1.7,4.872,-5.96647920544591E-16));
#8536=CARTESIAN_POINT('Origin',(1.7,6.42939569552361E-16,0.));
#8537=CARTESIAN_POINT('',(-1.7,4.872,-5.96647920544591E-16));
#8538=CARTESIAN_POINT('',(-1.8,4.872,-5.96647920544591E-16));
#8539=CARTESIAN_POINT('Origin',(-1.7,1.83697019872105E-17,0.));
#8540=CARTESIAN_POINT('Origin',(-1.8,0.,0.));
#8541=CARTESIAN_POINT('',(1.955,-4.8,5.90585918888811E-16));
#8542=CARTESIAN_POINT('',(1.955,4.8,-5.87830463590729E-16));
#8543=CARTESIAN_POINT('Origin',(1.955,6.89782309619747E-16,0.));
#8544=CARTESIAN_POINT('Origin',(1.955,6.89782309619747E-16,0.));
#8545=CARTESIAN_POINT('',(1.7,4.8,-5.87830463590729E-16));
#8546=CARTESIAN_POINT('',(-1.8,4.8,-5.87830463590729E-16));
#8547=CARTESIAN_POINT('Origin',(1.7,6.42939569552361E-16,0.));
#8548=CARTESIAN_POINT('Origin',(1.955,6.89782309619747E-16,0.));
#8549=CARTESIAN_POINT('',(2.,-4.845,-5.93341374186893E-16));
#8550=CARTESIAN_POINT('',(1.955,-4.8,-5.87830463590729E-16));
#8551=CARTESIAN_POINT('Origin',(2.,6.98048675513991E-16,0.));
#8552=CARTESIAN_POINT('Origin',(1.8,8.67361737988404E-16,0.));
#8553=CARTESIAN_POINT('',(1.8,6.,-7.34788079488412E-16));
#8554=CARTESIAN_POINT('Origin',(1.8,6.61309271539571E-16,0.));
#8555=CARTESIAN_POINT('',(2.,5.8,-7.10295143505465E-16));
#8556=CARTESIAN_POINT('Origin',(1.8,5.8,-7.10295143505465E-16));
#8557=CARTESIAN_POINT('Origin',(2.,6.98048675513991E-16,0.));
#8558=CARTESIAN_POINT('Origin',(-1.8,0.,0.));
#8559=CARTESIAN_POINT('',(-1.8,6.,-7.34788079488412E-16));
#8560=CARTESIAN_POINT('Origin',(-1.8,2.02467570659351E-31,0.));
#8561=CARTESIAN_POINT('',(-1.8,6.,-7.34788079488412E-16));
#8562=CARTESIAN_POINT('Origin',(-1.8,0.,0.));
#8563=CARTESIAN_POINT('',(-2.,5.8,-7.10295143505465E-16));
#8564=CARTESIAN_POINT('Origin',(-2.,-3.67394039744204E-17,0.));
#8565=CARTESIAN_POINT('Origin',(-1.8,5.8,-7.10295143505465E-16));
#8566=CARTESIAN_POINT('Origin',(-2.,-3.67394039744204E-17,0.));
#8567=CARTESIAN_POINT('',(-2.,4.845,-5.93341374186893E-16));
#8568=CARTESIAN_POINT('',(-2.,4.845,-5.93341374186893E-16));
#8569=CARTESIAN_POINT('Origin',(-2.,-3.67394039744204E-17,0.));
#8570=CARTESIAN_POINT('Origin',(-2.,5.8,0.));
#8571=CARTESIAN_POINT('Origin',(2.,5.8,0.));
#8572=CARTESIAN_POINT('Origin',(1.7,4.8,0.));
#8573=CARTESIAN_POINT('Origin',(-1.7,4.8,0.));
#8574=CARTESIAN_POINT('Origin',(-1.955,-2.84730380801757E-17,0.));
#8575=CARTESIAN_POINT('',(-1.955,3.1184375,3.81898450271607E-16));
#8576=CARTESIAN_POINT('',(-1.955,-3.1184375,-3.81898450271607E-16));
#8577=CARTESIAN_POINT('Origin',(-1.955,-2.84730380801757E-17,0.));
#8578=CARTESIAN_POINT('',(-2.,-3.0734375,-3.76387539675444E-16));
#8579=CARTESIAN_POINT('',(-1.955,-3.1184375,-3.81898450271607E-16));
#8580=CARTESIAN_POINT('Origin',(-2.,-3.67394039744204E-17,0.));
#8581=CARTESIAN_POINT('Origin',(-1.955,-2.84730380801757E-17,0.));
#8582=CARTESIAN_POINT('Origin',(-1.8,0.,0.));
#8583=CARTESIAN_POINT('',(-1.7890625,3.1184375,-3.81898450271607E-16));
#8584=CARTESIAN_POINT('',(-1.8,3.1184375,-3.81898450271607E-16));
#8585=CARTESIAN_POINT('Origin',(-1.7890625,2.00918615485137E-18,0.));
#8586=CARTESIAN_POINT('Origin',(-1.7890625,0.,0.));
#8587=CARTESIAN_POINT('',(-1.6625,3.2,-3.91886975727153E-16));
#8588=CARTESIAN_POINT('Origin',(-1.7890625,3.25741379310345,-3.98918137522258E-16));
#8589=CARTESIAN_POINT('Origin',(-1.6625,2.52583402324144E-17,0.));
#8590=CARTESIAN_POINT('Origin',(-1.8,0.,0.));
#8591=CARTESIAN_POINT('',(-1.6625,3.272,-4.00704432681014E-16));
#8592=CARTESIAN_POINT('Origin',(-1.6625,2.52583402324144E-17,0.));
#8593=CARTESIAN_POINT('',(1.6625,3.272,-4.00704432681014E-16));
#8594=CARTESIAN_POINT('',(-1.8,3.272,-4.00704432681014E-16));
#8595=CARTESIAN_POINT('Origin',(1.6625,6.36050931307157E-16,0.));
#8596=CARTESIAN_POINT('Origin',(1.7890625,8.67361737988404E-16,0.));
#8597=CARTESIAN_POINT('',(1.6625,3.2,-3.91886975727153E-16));
#8598=CARTESIAN_POINT('Origin',(1.6625,6.36050931307157E-16,0.));
#8599=CARTESIAN_POINT('',(1.7890625,3.1184375,-3.81898450271607E-16));
#8600=CARTESIAN_POINT('Origin',(1.7890625,3.25741379310345,-3.98918137522258E-16));
#8601=CARTESIAN_POINT('Origin',(1.7890625,6.5930008538472E-16,0.));
#8602=CARTESIAN_POINT('Origin',(-1.8,0.,0.));
#8603=CARTESIAN_POINT('',(1.955,3.1184375,-3.81898450271607E-16));
#8604=CARTESIAN_POINT('',(-1.8,3.1184375,-3.81898450271607E-16));
#8605=CARTESIAN_POINT('Origin',(1.955,6.89782309619747E-16,0.));
#8606=CARTESIAN_POINT('Origin',(2.,6.98048675513991E-16,0.));
#8607=CARTESIAN_POINT('',(2.,3.0734375,-3.76387539675444E-16));
#8608=CARTESIAN_POINT('',(2.,3.0734375,-3.76387539675444E-16));
#8609=CARTESIAN_POINT('Origin',(2.,6.98048675513991E-16,0.));
#8610=CARTESIAN_POINT('Origin',(1.8,8.67361737988404E-16,0.));
#8611=CARTESIAN_POINT('',(2.,2.2,-2.69422295812418E-16));
#8612=CARTESIAN_POINT('Origin',(2.,6.98048675513991E-16,0.));
#8613=CARTESIAN_POINT('',(1.8,2.,-2.44929359829471E-16));
#8614=CARTESIAN_POINT('Origin',(1.8,2.2,-2.69422295812418E-16));
#8615=CARTESIAN_POINT('Origin',(1.8,6.61309271539571E-16,0.));
#8616=CARTESIAN_POINT('Origin',(-1.8,0.,0.));
#8617=CARTESIAN_POINT('',(-1.8,2.,-2.44929359829471E-16));
#8618=CARTESIAN_POINT('',(-1.8,2.,-2.44929359829471E-16));
#8619=CARTESIAN_POINT('Origin',(-1.8,1.86988015034452E-31,0.));
#8620=CARTESIAN_POINT('Origin',(-1.8,0.,0.));
#8621=CARTESIAN_POINT('',(-2.,2.2,-2.69422295812418E-16));
#8622=CARTESIAN_POINT('Origin',(-1.8,2.2,-2.69422295812418E-16));
#8623=CARTESIAN_POINT('Origin',(-2.,-3.67394039744205E-17,0.));
#8624=CARTESIAN_POINT('Origin',(2.,2.2,0.));
#8625=CARTESIAN_POINT('Origin',(1.6625,3.272,0.));
#8626=CARTESIAN_POINT('Origin',(-1.6625,3.2,0.));
#8627=CARTESIAN_POINT('Origin',(-2.,2.2,0.));
#8628=CARTESIAN_POINT('Origin',(-1.8,0.,0.));
#8629=CARTESIAN_POINT('',(1.95,3.2,-3.91886975727153E-16));
#8630=CARTESIAN_POINT('Origin',(1.95,6.88863824520387E-16,0.));
#8631=CARTESIAN_POINT('',(1.85,3.2,-3.91886975727153E-16));
#8632=CARTESIAN_POINT('',(-1.8,3.2,-3.91886975727153E-16));
#8633=CARTESIAN_POINT('Origin',(1.85,6.70494122533176E-16,0.));
#8634=CARTESIAN_POINT('Origin',(1.86,8.67361737988404E-16,0.));
#8635=CARTESIAN_POINT('',(1.905,4.22108058265378,-5.16933282449E-16));
#8636=CARTESIAN_POINT('Origin',(1.905,6.80597458626142E-16,0.));
#8637=CARTESIAN_POINT('',(1.95,4.14313829631318,-5.07388105300476E-16));
#8638=CARTESIAN_POINT('Origin',(1.86,4.14313829631318,-5.07388105300475E-16));
#8639=CARTESIAN_POINT('Origin',(1.95,6.88863824520387E-16,0.));
#8640=CARTESIAN_POINT('Origin',(1.65333333333334,6.34367041958329E-16,0.));
#8641=CARTESIAN_POINT('',(1.65333333333334,4.36638040039984,-5.3472737812094E-16));
#8642=CARTESIAN_POINT('Origin',(1.65333333333334,6.34367041958329E-16,0.));
#8643=CARTESIAN_POINT('',(1.65333333333334,4.36638040039984,-5.3472737812094E-16));
#8644=CARTESIAN_POINT('Origin',(1.66333333333334,8.67361737988404E-16,0.));
#8645=CARTESIAN_POINT('',(1.64333333333333,4.38370090847553,-5.3684852859839E-16));
#8646=CARTESIAN_POINT('Origin',(1.64333333333334,6.32530071759608E-16,0.));
#8647=CARTESIAN_POINT('Origin',(1.66333333333334,4.38370090847553,-5.3684852859839E-16));
#8648=CARTESIAN_POINT('Origin',(1.76333333333333,8.67361737988404E-16,0.));
#8649=CARTESIAN_POINT('',(1.86725638178747,4.64,-5.68236114804372E-16));
#8650=CARTESIAN_POINT('Origin',(1.86725638178747,6.73664068441309E-16,0.));
#8651=CARTESIAN_POINT('',(1.64333333333333,4.58,-5.60888234009488E-16));
#8652=CARTESIAN_POINT('Origin',(1.76333333333333,4.58,-5.60888234009488E-16));
#8653=CARTESIAN_POINT('Origin',(1.64333333333334,6.32530071759608E-16,0.));
#8654=CARTESIAN_POINT('Origin',(1.90725638178747,6.81011949236193E-16,0.));
#8655=CARTESIAN_POINT('',(1.90725638178747,4.57071796769724,-5.59751512894572E-16));
#8656=CARTESIAN_POINT('Origin',(1.90725638178747,6.81011949236193E-16,0.));
#8657=CARTESIAN_POINT('',(1.90725638178747,4.57071796769724,-5.59751512894572E-16));
#8658=CARTESIAN_POINT('Origin',(1.80333333333334,8.67361737988404E-16,0.));
#8659=CARTESIAN_POINT('',(1.80333333333334,4.39071796769724,-5.3770787050992E-16));
#8660=CARTESIAN_POINT('Origin',(1.80333333333334,6.61921594939145E-16,0.));
#8661=CARTESIAN_POINT('Origin',(1.80333333333334,4.51071796769724,-5.52403632099688E-16));
#8662=CARTESIAN_POINT('Origin',(1.80333333333334,8.67361737988404E-16,0.));
#8663=CARTESIAN_POINT('',(1.99385892216591,4.62071796769724,-5.65874746890309E-16));
#8664=CARTESIAN_POINT('Origin',(1.99385892216591,6.96920577817067E-16,0.));
#8665=CARTESIAN_POINT('',(1.80333333333334,4.29071796769724,-5.25461402518447E-16));
#8666=CARTESIAN_POINT('Origin',(1.80333333333334,4.51071796769724,-5.52403632099688E-16));
#8667=CARTESIAN_POINT('Origin',(1.80333333333334,6.61921594939145E-16,0.));
#8668=CARTESIAN_POINT('Origin',(1.99385892216591,6.96920577817067E-16,0.));
#8669=CARTESIAN_POINT('',(1.95385892216591,4.69,-5.74359348800109E-16));
#8670=CARTESIAN_POINT('Origin',(1.95385892216591,6.89572697022182E-16,0.));
#8671=CARTESIAN_POINT('',(1.99385892216591,4.62071796769724,-5.65874746890309E-16));
#8672=CARTESIAN_POINT('Origin',(1.76333333333333,8.67361737988404E-16,0.));
#8673=CARTESIAN_POINT('',(1.54333333333334,4.58,-5.60888234009488E-16));
#8674=CARTESIAN_POINT('Origin',(1.54333333333334,6.14160369772398E-16,0.));
#8675=CARTESIAN_POINT('Origin',(1.76333333333333,4.58,-5.60888234009488E-16));
#8676=CARTESIAN_POINT('Origin',(1.66333333333334,8.67361737988404E-16,0.));
#8677=CARTESIAN_POINT('',(1.60333333333334,4.27977786002139,-5.24121625733691E-16));
#8678=CARTESIAN_POINT('Origin',(1.60333333333334,6.25182190964724E-16,0.));
#8679=CARTESIAN_POINT('',(1.54333333333333,4.38370090847553,-5.3684852859839E-16));
#8680=CARTESIAN_POINT('Origin',(1.66333333333334,4.38370090847553,-5.3684852859839E-16));
#8681=CARTESIAN_POINT('Origin',(1.54333333333334,6.14160369772398E-16,0.));
#8682=CARTESIAN_POINT('Origin',(1.60333333333334,6.25182190964724E-16,0.));
#8683=CARTESIAN_POINT('',(1.85,4.13736479362129,-5.06681055141326E-16));
#8684=CARTESIAN_POINT('Origin',(1.85,6.70494122533176E-16,0.));
#8685=CARTESIAN_POINT('',(1.60333333333334,4.27977786002139,-5.2412162573369E-16));
#8686=CARTESIAN_POINT('Origin',(1.85,4.14313829631318,0.));
#8687=CARTESIAN_POINT('Origin',(1.54333333333334,4.58,0.));
#8688=CARTESIAN_POINT('Origin',(1.80333333333334,4.29071796769724,0.));
#8689=CARTESIAN_POINT('Origin',(1.64333333333334,4.58,0.));
#8690=CARTESIAN_POINT('Origin',(1.95,4.14313829631318,0.));
#8691=CARTESIAN_POINT('Origin',(1.8,0.,0.));
#8692=CARTESIAN_POINT('',(-1.95,3.2,3.91886975727153E-16));
#8693=CARTESIAN_POINT('Origin',(-1.95,6.88863824520387E-16,0.));
#8694=CARTESIAN_POINT('',(-1.85,3.2,3.91886975727153E-16));
#8695=CARTESIAN_POINT('',(1.8,3.2,3.91886975727153E-16));
#8696=CARTESIAN_POINT('Origin',(-1.85,6.70494122533176E-16,0.));
#8697=CARTESIAN_POINT('Origin',(-1.86,8.67361737988404E-16,0.));
#8698=CARTESIAN_POINT('',(-1.905,4.22108058265378,5.16933282449E-16));
#8699=CARTESIAN_POINT('Origin',(-1.905,6.80597458626142E-16,0.));
#8700=CARTESIAN_POINT('',(-1.95,4.14313829631318,5.07388105300476E-16));
#8701=CARTESIAN_POINT('Origin',(-1.86,4.14313829631318,5.07388105300475E-16));
#8702=CARTESIAN_POINT('Origin',(-1.95,6.88863824520387E-16,0.));
#8703=CARTESIAN_POINT('Origin',(-1.65333333333334,6.34367041958329E-16,
0.));
#8704=CARTESIAN_POINT('',(-1.65333333333334,4.36638040039984,5.3472737812094E-16));
#8705=CARTESIAN_POINT('Origin',(-1.65333333333334,6.34367041958329E-16,
0.));
#8706=CARTESIAN_POINT('',(-1.65333333333334,4.36638040039984,5.3472737812094E-16));
#8707=CARTESIAN_POINT('Origin',(-1.66333333333334,8.67361737988404E-16,
0.));
#8708=CARTESIAN_POINT('',(-1.64333333333333,4.38370090847553,5.3684852859839E-16));
#8709=CARTESIAN_POINT('Origin',(-1.64333333333334,6.32530071759608E-16,
0.));
#8710=CARTESIAN_POINT('Origin',(-1.66333333333334,4.38370090847553,5.3684852859839E-16));
#8711=CARTESIAN_POINT('Origin',(-1.76333333333333,8.67361737988404E-16,
0.));
#8712=CARTESIAN_POINT('',(-1.86725638178747,4.64,5.68236114804372E-16));
#8713=CARTESIAN_POINT('Origin',(-1.86725638178747,6.73664068441309E-16,
0.));
#8714=CARTESIAN_POINT('',(-1.64333333333333,4.58,5.60888234009488E-16));
#8715=CARTESIAN_POINT('Origin',(-1.76333333333333,4.58,5.60888234009488E-16));
#8716=CARTESIAN_POINT('Origin',(-1.64333333333334,6.32530071759608E-16,
0.));
#8717=CARTESIAN_POINT('Origin',(-1.90725638178747,6.81011949236193E-16,
0.));
#8718=CARTESIAN_POINT('',(-1.90725638178747,4.57071796769724,5.59751512894572E-16));
#8719=CARTESIAN_POINT('Origin',(-1.90725638178747,6.81011949236193E-16,
0.));
#8720=CARTESIAN_POINT('',(-1.90725638178747,4.57071796769724,5.59751512894572E-16));
#8721=CARTESIAN_POINT('Origin',(-1.80333333333334,8.67361737988404E-16,
0.));
#8722=CARTESIAN_POINT('',(-1.80333333333334,4.39071796769724,5.3770787050992E-16));
#8723=CARTESIAN_POINT('Origin',(-1.80333333333334,6.61921594939145E-16,
0.));
#8724=CARTESIAN_POINT('Origin',(-1.80333333333334,4.51071796769724,5.52403632099688E-16));
#8725=CARTESIAN_POINT('Origin',(-1.80333333333334,8.67361737988404E-16,
0.));
#8726=CARTESIAN_POINT('',(-1.99385892216591,4.62071796769724,5.65874746890309E-16));
#8727=CARTESIAN_POINT('Origin',(-1.99385892216591,6.96920577817067E-16,
0.));
#8728=CARTESIAN_POINT('',(-1.80333333333334,4.29071796769724,5.25461402518447E-16));
#8729=CARTESIAN_POINT('Origin',(-1.80333333333334,4.51071796769724,5.52403632099688E-16));
#8730=CARTESIAN_POINT('Origin',(-1.80333333333334,6.61921594939145E-16,
0.));
#8731=CARTESIAN_POINT('Origin',(-1.99385892216591,6.96920577817067E-16,
0.));
#8732=CARTESIAN_POINT('',(-1.95385892216591,4.69,5.74359348800109E-16));
#8733=CARTESIAN_POINT('Origin',(-1.95385892216591,6.89572697022182E-16,
0.));
#8734=CARTESIAN_POINT('',(-1.99385892216591,4.62071796769724,5.65874746890309E-16));
#8735=CARTESIAN_POINT('Origin',(-1.76333333333333,8.67361737988404E-16,
0.));
#8736=CARTESIAN_POINT('',(-1.54333333333334,4.58,5.60888234009488E-16));
#8737=CARTESIAN_POINT('Origin',(-1.54333333333334,6.14160369772398E-16,
0.));
#8738=CARTESIAN_POINT('Origin',(-1.76333333333333,4.58,5.60888234009488E-16));
#8739=CARTESIAN_POINT('Origin',(-1.66333333333334,8.67361737988404E-16,
0.));
#8740=CARTESIAN_POINT('',(-1.60333333333334,4.27977786002139,5.24121625733691E-16));
#8741=CARTESIAN_POINT('Origin',(-1.60333333333334,6.25182190964724E-16,
0.));
#8742=CARTESIAN_POINT('',(-1.54333333333333,4.38370090847553,5.3684852859839E-16));
#8743=CARTESIAN_POINT('Origin',(-1.66333333333334,4.38370090847553,5.3684852859839E-16));
#8744=CARTESIAN_POINT('Origin',(-1.54333333333334,6.14160369772398E-16,
0.));
#8745=CARTESIAN_POINT('Origin',(-1.60333333333334,6.25182190964724E-16,
0.));
#8746=CARTESIAN_POINT('',(-1.85,4.13736479362129,5.06681055141326E-16));
#8747=CARTESIAN_POINT('Origin',(-1.85,6.70494122533176E-16,0.));
#8748=CARTESIAN_POINT('',(-1.60333333333334,4.27977786002139,5.2412162573369E-16));
#8749=CARTESIAN_POINT('Origin',(-1.85,4.14313829631318,0.));
#8750=CARTESIAN_POINT('Origin',(-1.54333333333334,4.58,0.));
#8751=CARTESIAN_POINT('Origin',(-1.80333333333334,4.29071796769724,0.));
#8752=CARTESIAN_POINT('Origin',(-1.64333333333334,4.58,0.));
#8753=CARTESIAN_POINT('Origin',(-1.95,4.14313829631318,0.));
#8769=UNCERTAINTY_MEASURE_WITH_UNIT(LENGTH_MEASURE(0.01),#8780,
'DISTANCE_ACCURACY_VALUE',
'Maximum model space distance between geometric entities at asserted c
onnectivities');
#8770=UNCERTAINTY_MEASURE_WITH_UNIT(LENGTH_MEASURE(0.01),#8780,
'DISTANCE_ACCURACY_VALUE',
'Maximum model space distance between geometric entities at asserted c
onnectivities');
#8778=(
GEOMETRIC_REPRESENTATION_CONTEXT(3)
GLOBAL_UNCERTAINTY_ASSIGNED_CONTEXT((#8769))
GLOBAL_UNIT_ASSIGNED_CONTEXT((#8780,#8782,#8783))
REPRESENTATION_CONTEXT('','3D')
);
#8779=(
GEOMETRIC_REPRESENTATION_CONTEXT(3)
GLOBAL_UNCERTAINTY_ASSIGNED_CONTEXT((#8770))
GLOBAL_UNIT_ASSIGNED_CONTEXT((#8780,#8782,#8783))
REPRESENTATION_CONTEXT('','3D')
);
#8780=(
LENGTH_UNIT()
NAMED_UNIT(*)
SI_UNIT(.MILLI.,.METRE.)
);
#8782=(
NAMED_UNIT(*)
PLANE_ANGLE_UNIT()
SI_UNIT($,.RADIAN.)
);
#8783=(
NAMED_UNIT(*)
SI_UNIT($,.STERADIAN.)
SOLID_ANGLE_UNIT()
);
#8791=SHAPE_DEFINITION_REPRESENTATION(#8799,#8815);
#8799=PRODUCT_DEFINITION_SHAPE('',$,#8824);
#8815=SHAPE_REPRESENTATION('',(#5571),#8778);
#8816=PRODUCT_DEFINITION_CONTEXT('part definition',#8842,'design');
#8824=PRODUCT_DEFINITION('Bearing_01','Bearing_01',#8832,#8816);
#8832=PRODUCT_DEFINITION_FORMATION('',$,#8851);
#8842=APPLICATION_CONTEXT(
'Core Data for Automotive Mechanical Design Process');
#8843=PRODUCT_CONTEXT('part definition',#8842,'mechanical');
#8851=PRODUCT('Bearing_01','Bearing_01',$,(#8843));
#8856=PRESENTATION_STYLE_ASSIGNMENT((#8861));
#8861=SURFACE_STYLE_USAGE(.BOTH.,#8866);
#8866=SURFACE_SIDE_STYLE('',(#8871));
#8871=SURFACE_STYLE_FILL_AREA(#8876);
#8876=FILL_AREA_STYLE('Opaque(160,160,160)',(#8881));
#8881=FILL_AREA_STYLE_COLOUR('Opaque(160,160,160)',#8886);
#8886=COLOUR_RGB('Opaque(160,160,160)', 0.72549020, 0.75294118, 0.79215686);
ENDSEC;
END-ISO-10303-21;
